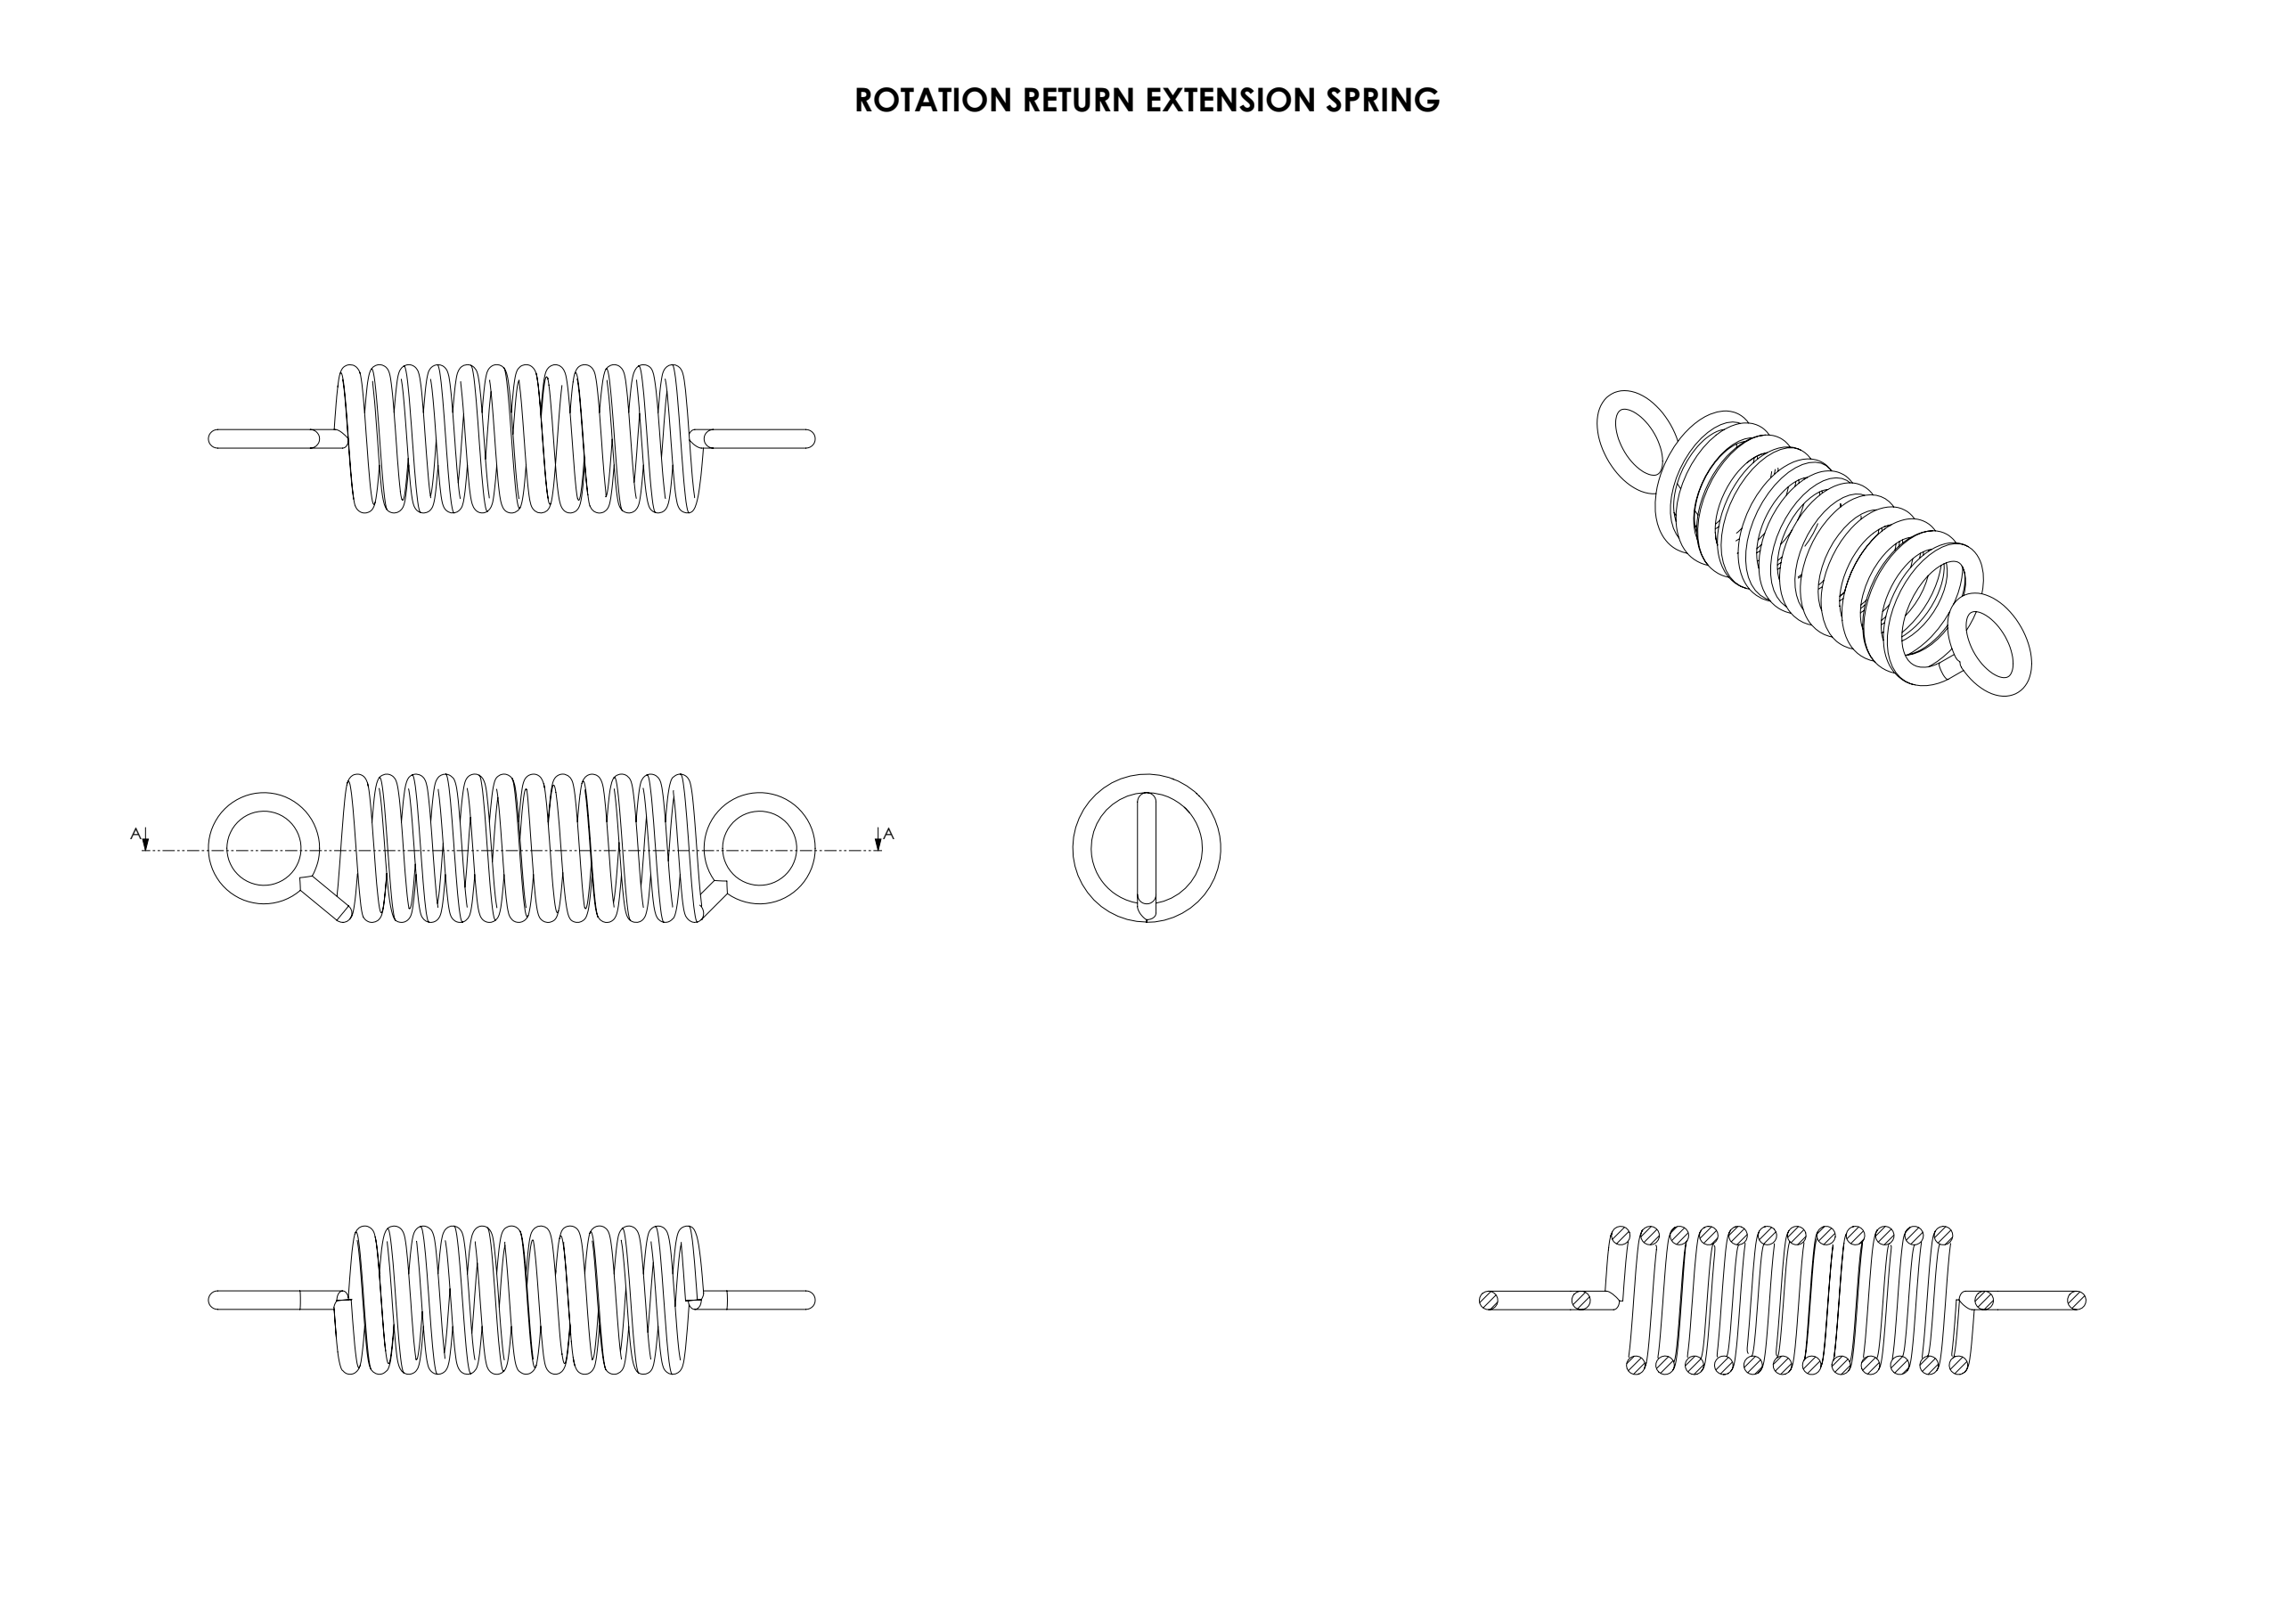
ISO-10303-21;
HEADER;
/* Generated by software containing ST-Developer
 * from STEP Tools, Inc. (www.steptools.com) 
 */

FILE_DESCRIPTION(
/* description */ (''),
/* implementation_level */ '2;1');

FILE_NAME(
/* name */ '16_Rotation_Return_Extension_Spring.step',
/* time_stamp */ '2026-10-21T01:56:51-07:00',
/* author */ (''),
/* organization */ (''),
/* preprocessor_version */ 'ST-DEVELOPER v20.2',
/* originating_system */ 'Autodesk Translation Framework v15.15.0.0',
/* authorisation */ '');

FILE_SCHEMA (('AUTOMOTIVE_DESIGN { 1 0 10303 214 3 1 1 }'));
ENDSEC;

DATA;
#10=MECHANICAL_DESIGN_GEOMETRIC_PRESENTATION_REPRESENTATION('',(#274),#82384);
#157=TOROIDAL_SURFACE('',#31771,2.,0.4);
#158=TOROIDAL_SURFACE('',#31779,2.,0.4);
#236=SHAPE_REPRESENTATION_RELATIONSHIP('SRR','None',#82470,#255);
#255=ADVANCED_BREP_SHAPE_REPRESENTATION('',(#293),#82369);
#274=STYLED_ITEM('',(#82631),#293);
#293=MANIFOLD_SOLID_BREP('Body1',#30665);
#418=B_SPLINE_SURFACE_WITH_KNOTS('',3,3,((#45016,#45017,#45018,#45019,#45020,
#45021,#45022,#45023,#45024,#45025,#45026,#45027,#45028,#45029,#45030,#45031,
#45032,#45033,#45034,#45035,#45036,#45037,#45038,#45039,#45040,#45041,#45042,
#45043,#45044,#45045,#45046,#45047,#45048,#45049,#45050,#45051,#45052,#45053,
#45054,#45055,#45056,#45057,#45058,#45059,#45060,#45061,#45062,#45063,#45064,
#45065,#45066,#45067,#45068,#45069,#45070,#45071,#45072,#45073,#45074,#45075,
#45076,#45077,#45078,#45079,#45080,#45081,#45082,#45083,#45084,#45085,#45086,
#45087,#45088,#45089,#45090,#45091,#45092,#45093,#45094,#45095,#45096,#45097,
#45098,#45099,#45100,#45101,#45102,#45103,#45104,#45105,#45106,#45107,#45108,
#45109,#45110,#45111,#45112,#45113,#45114,#45115,#45116,#45117,#45118,#45119,
#45120,#45121,#45122,#45123,#45124,#45125,#45126,#45127,#45128,#45129,#45130,
#45131,#45132,#45133,#45134,#45135,#45136,#45137,#45138,#45139,#45140,#45141,
#45142),(#45143,#45144,#45145,#45146,#45147,#45148,#45149,#45150,#45151,
#45152,#45153,#45154,#45155,#45156,#45157,#45158,#45159,#45160,#45161,#45162,
#45163,#45164,#45165,#45166,#45167,#45168,#45169,#45170,#45171,#45172,#45173,
#45174,#45175,#45176,#45177,#45178,#45179,#45180,#45181,#45182,#45183,#45184,
#45185,#45186,#45187,#45188,#45189,#45190,#45191,#45192,#45193,#45194,#45195,
#45196,#45197,#45198,#45199,#45200,#45201,#45202,#45203,#45204,#45205,#45206,
#45207,#45208,#45209,#45210,#45211,#45212,#45213,#45214,#45215,#45216,#45217,
#45218,#45219,#45220,#45221,#45222,#45223,#45224,#45225,#45226,#45227,#45228,
#45229,#45230,#45231,#45232,#45233,#45234,#45235,#45236,#45237,#45238,#45239,
#45240,#45241,#45242,#45243,#45244,#45245,#45246,#45247,#45248,#45249,#45250,
#45251,#45252,#45253,#45254,#45255,#45256,#45257,#45258,#45259,#45260,#45261,
#45262,#45263,#45264,#45265,#45266,#45267,#45268,#45269),(#45270,#45271,
#45272,#45273,#45274,#45275,#45276,#45277,#45278,#45279,#45280,#45281,#45282,
#45283,#45284,#45285,#45286,#45287,#45288,#45289,#45290,#45291,#45292,#45293,
#45294,#45295,#45296,#45297,#45298,#45299,#45300,#45301,#45302,#45303,#45304,
#45305,#45306,#45307,#45308,#45309,#45310,#45311,#45312,#45313,#45314,#45315,
#45316,#45317,#45318,#45319,#45320,#45321,#45322,#45323,#45324,#45325,#45326,
#45327,#45328,#45329,#45330,#45331,#45332,#45333,#45334,#45335,#45336,#45337,
#45338,#45339,#45340,#45341,#45342,#45343,#45344,#45345,#45346,#45347,#45348,
#45349,#45350,#45351,#45352,#45353,#45354,#45355,#45356,#45357,#45358,#45359,
#45360,#45361,#45362,#45363,#45364,#45365,#45366,#45367,#45368,#45369,#45370,
#45371,#45372,#45373,#45374,#45375,#45376,#45377,#45378,#45379,#45380,#45381,
#45382,#45383,#45384,#45385,#45386,#45387,#45388,#45389,#45390,#45391,#45392,
#45393,#45394,#45395,#45396),(#45397,#45398,#45399,#45400,#45401,#45402,
#45403,#45404,#45405,#45406,#45407,#45408,#45409,#45410,#45411,#45412,#45413,
#45414,#45415,#45416,#45417,#45418,#45419,#45420,#45421,#45422,#45423,#45424,
#45425,#45426,#45427,#45428,#45429,#45430,#45431,#45432,#45433,#45434,#45435,
#45436,#45437,#45438,#45439,#45440,#45441,#45442,#45443,#45444,#45445,#45446,
#45447,#45448,#45449,#45450,#45451,#45452,#45453,#45454,#45455,#45456,#45457,
#45458,#45459,#45460,#45461,#45462,#45463,#45464,#45465,#45466,#45467,#45468,
#45469,#45470,#45471,#45472,#45473,#45474,#45475,#45476,#45477,#45478,#45479,
#45480,#45481,#45482,#45483,#45484,#45485,#45486,#45487,#45488,#45489,#45490,
#45491,#45492,#45493,#45494,#45495,#45496,#45497,#45498,#45499,#45500,#45501,
#45502,#45503,#45504,#45505,#45506,#45507,#45508,#45509,#45510,#45511,#45512,
#45513,#45514,#45515,#45516,#45517,#45518,#45519,#45520,#45521,#45522,#45523),
(#45524,#45525,#45526,#45527,#45528,#45529,#45530,#45531,#45532,#45533,
#45534,#45535,#45536,#45537,#45538,#45539,#45540,#45541,#45542,#45543,#45544,
#45545,#45546,#45547,#45548,#45549,#45550,#45551,#45552,#45553,#45554,#45555,
#45556,#45557,#45558,#45559,#45560,#45561,#45562,#45563,#45564,#45565,#45566,
#45567,#45568,#45569,#45570,#45571,#45572,#45573,#45574,#45575,#45576,#45577,
#45578,#45579,#45580,#45581,#45582,#45583,#45584,#45585,#45586,#45587,#45588,
#45589,#45590,#45591,#45592,#45593,#45594,#45595,#45596,#45597,#45598,#45599,
#45600,#45601,#45602,#45603,#45604,#45605,#45606,#45607,#45608,#45609,#45610,
#45611,#45612,#45613,#45614,#45615,#45616,#45617,#45618,#45619,#45620,#45621,
#45622,#45623,#45624,#45625,#45626,#45627,#45628,#45629,#45630,#45631,#45632,
#45633,#45634,#45635,#45636,#45637,#45638,#45639,#45640,#45641,#45642,#45643,
#45644,#45645,#45646,#45647,#45648,#45649,#45650),(#45651,#45652,#45653,
#45654,#45655,#45656,#45657,#45658,#45659,#45660,#45661,#45662,#45663,#45664,
#45665,#45666,#45667,#45668,#45669,#45670,#45671,#45672,#45673,#45674,#45675,
#45676,#45677,#45678,#45679,#45680,#45681,#45682,#45683,#45684,#45685,#45686,
#45687,#45688,#45689,#45690,#45691,#45692,#45693,#45694,#45695,#45696,#45697,
#45698,#45699,#45700,#45701,#45702,#45703,#45704,#45705,#45706,#45707,#45708,
#45709,#45710,#45711,#45712,#45713,#45714,#45715,#45716,#45717,#45718,#45719,
#45720,#45721,#45722,#45723,#45724,#45725,#45726,#45727,#45728,#45729,#45730,
#45731,#45732,#45733,#45734,#45735,#45736,#45737,#45738,#45739,#45740,#45741,
#45742,#45743,#45744,#45745,#45746,#45747,#45748,#45749,#45750,#45751,#45752,
#45753,#45754,#45755,#45756,#45757,#45758,#45759,#45760,#45761,#45762,#45763,
#45764,#45765,#45766,#45767,#45768,#45769,#45770,#45771,#45772,#45773,#45774,
#45775,#45776,#45777),(#45778,#45779,#45780,#45781,#45782,#45783,#45784,
#45785,#45786,#45787,#45788,#45789,#45790,#45791,#45792,#45793,#45794,#45795,
#45796,#45797,#45798,#45799,#45800,#45801,#45802,#45803,#45804,#45805,#45806,
#45807,#45808,#45809,#45810,#45811,#45812,#45813,#45814,#45815,#45816,#45817,
#45818,#45819,#45820,#45821,#45822,#45823,#45824,#45825,#45826,#45827,#45828,
#45829,#45830,#45831,#45832,#45833,#45834,#45835,#45836,#45837,#45838,#45839,
#45840,#45841,#45842,#45843,#45844,#45845,#45846,#45847,#45848,#45849,#45850,
#45851,#45852,#45853,#45854,#45855,#45856,#45857,#45858,#45859,#45860,#45861,
#45862,#45863,#45864,#45865,#45866,#45867,#45868,#45869,#45870,#45871,#45872,
#45873,#45874,#45875,#45876,#45877,#45878,#45879,#45880,#45881,#45882,#45883,
#45884,#45885,#45886,#45887,#45888,#45889,#45890,#45891,#45892,#45893,#45894,
#45895,#45896,#45897,#45898,#45899,#45900,#45901,#45902,#45903,#45904),
(#45905,#45906,#45907,#45908,#45909,#45910,#45911,#45912,#45913,#45914,
#45915,#45916,#45917,#45918,#45919,#45920,#45921,#45922,#45923,#45924,#45925,
#45926,#45927,#45928,#45929,#45930,#45931,#45932,#45933,#45934,#45935,#45936,
#45937,#45938,#45939,#45940,#45941,#45942,#45943,#45944,#45945,#45946,#45947,
#45948,#45949,#45950,#45951,#45952,#45953,#45954,#45955,#45956,#45957,#45958,
#45959,#45960,#45961,#45962,#45963,#45964,#45965,#45966,#45967,#45968,#45969,
#45970,#45971,#45972,#45973,#45974,#45975,#45976,#45977,#45978,#45979,#45980,
#45981,#45982,#45983,#45984,#45985,#45986,#45987,#45988,#45989,#45990,#45991,
#45992,#45993,#45994,#45995,#45996,#45997,#45998,#45999,#46000,#46001,#46002,
#46003,#46004,#46005,#46006,#46007,#46008,#46009,#46010,#46011,#46012,#46013,
#46014,#46015,#46016,#46017,#46018,#46019,#46020,#46021,#46022,#46023,#46024,
#46025,#46026,#46027,#46028,#46029,#46030,#46031),(#46032,#46033,#46034,
#46035,#46036,#46037,#46038,#46039,#46040,#46041,#46042,#46043,#46044,#46045,
#46046,#46047,#46048,#46049,#46050,#46051,#46052,#46053,#46054,#46055,#46056,
#46057,#46058,#46059,#46060,#46061,#46062,#46063,#46064,#46065,#46066,#46067,
#46068,#46069,#46070,#46071,#46072,#46073,#46074,#46075,#46076,#46077,#46078,
#46079,#46080,#46081,#46082,#46083,#46084,#46085,#46086,#46087,#46088,#46089,
#46090,#46091,#46092,#46093,#46094,#46095,#46096,#46097,#46098,#46099,#46100,
#46101,#46102,#46103,#46104,#46105,#46106,#46107,#46108,#46109,#46110,#46111,
#46112,#46113,#46114,#46115,#46116,#46117,#46118,#46119,#46120,#46121,#46122,
#46123,#46124,#46125,#46126,#46127,#46128,#46129,#46130,#46131,#46132,#46133,
#46134,#46135,#46136,#46137,#46138,#46139,#46140,#46141,#46142,#46143,#46144,
#46145,#46146,#46147,#46148,#46149,#46150,#46151,#46152,#46153,#46154,#46155,
#46156,#46157,#46158),(#46159,#46160,#46161,#46162,#46163,#46164,#46165,
#46166,#46167,#46168,#46169,#46170,#46171,#46172,#46173,#46174,#46175,#46176,
#46177,#46178,#46179,#46180,#46181,#46182,#46183,#46184,#46185,#46186,#46187,
#46188,#46189,#46190,#46191,#46192,#46193,#46194,#46195,#46196,#46197,#46198,
#46199,#46200,#46201,#46202,#46203,#46204,#46205,#46206,#46207,#46208,#46209,
#46210,#46211,#46212,#46213,#46214,#46215,#46216,#46217,#46218,#46219,#46220,
#46221,#46222,#46223,#46224,#46225,#46226,#46227,#46228,#46229,#46230,#46231,
#46232,#46233,#46234,#46235,#46236,#46237,#46238,#46239,#46240,#46241,#46242,
#46243,#46244,#46245,#46246,#46247,#46248,#46249,#46250,#46251,#46252,#46253,
#46254,#46255,#46256,#46257,#46258,#46259,#46260,#46261,#46262,#46263,#46264,
#46265,#46266,#46267,#46268,#46269,#46270,#46271,#46272,#46273,#46274,#46275,
#46276,#46277,#46278,#46279,#46280,#46281,#46282,#46283,#46284,#46285)),
 .UNSPECIFIED.,.T.,.F.,.F.,(4,1,1,1,1,1,1,4),(4,1,1,1,1,1,1,1,1,1,1,1,1,
1,1,1,1,1,1,1,1,1,1,1,1,1,1,1,1,1,1,1,1,1,1,1,1,1,1,1,1,1,1,1,1,1,1,1,1,
1,1,1,1,1,1,1,1,1,1,1,1,1,1,1,1,1,1,1,1,1,1,1,1,1,1,1,1,1,1,1,1,1,1,1,1,
1,1,1,1,1,1,1,1,1,1,1,1,1,1,1,1,1,1,1,1,1,1,1,1,1,1,1,1,1,1,1,1,1,1,1,1,
1,1,1,4),(-3.14159265358979,-2.24399475256414,-1.34639685153848,-0.448798950512828,
0.448798950512828,1.34639685153848,2.24399475256414,3.14159265358979),(0.,
0.00446428571428571,0.00892857142857143,0.0178571428571429,0.0267857142857143,
0.0357142857142857,0.0446428571428571,0.0535714285714286,0.0625,0.0714285714285714,
0.0803571428571428,0.0892857142857143,0.0982142857142857,0.107142857142857,
0.116071428571429,0.125,0.129464285714286,0.133928571428571,0.138392857142857,
0.142857142857143,0.151785714285714,0.160714285714286,0.169642857142857,
0.178571428571429,0.1875,0.196428571428571,0.205357142857143,0.214285714285714,
0.223214285714286,0.232142857142857,0.241071428571429,0.25,0.258928571428571,
0.267857142857143,0.276785714285714,0.285714285714286,0.294642857142857,
0.303571428571429,0.3125,0.321428571428571,0.330357142857143,0.339285714285714,
0.348214285714286,0.357142857142857,0.366071428571428,0.375,0.383928571428571,
0.392857142857143,0.401785714285714,0.410714285714286,0.419642857142857,
0.428571428571429,0.4375,0.446428571428571,0.455357142857143,0.464285714285714,
0.473214285714286,0.482142857142857,0.494047619047619,0.5,0.504464285714286,
0.508928571428571,0.517857142857143,0.526785714285714,0.535714285714286,
0.544642857142857,0.553571428571429,0.5625,0.571428571428571,0.580357142857143,
0.589285714285714,0.598214285714286,0.607142857142857,0.616071428571429,
0.625,0.633928571428571,0.642857142857143,0.647321428571428,0.651785714285714,
0.660714285714286,0.666666666666667,0.678571428571428,0.6796875,0.680803571428571,
0.6875,0.696428571428571,0.705357142857143,0.714285714285714,0.726190476190476,
0.735119047619047,0.738095238095238,0.75,0.761904761904762,0.76984126984127,
0.777777777777778,0.785714285714286,0.793650793650794,0.801587301587302,
0.809523809523809,0.81547619047619,0.821428571428571,0.827380952380952,
0.830357142857143,0.833333333333333,0.839285714285714,0.845238095238095,
0.851190476190476,0.857142857142857,0.866071428571429,0.875,0.883928571428571,
0.892857142857143,0.901785714285714,0.910714285714286,0.919642857142857,
0.928571428571429,0.9375,0.946428571428571,0.955357142857143,0.964285714285714,
0.973214285714286,0.982142857142857,0.991071428571429,0.995535714285714,
1.),.UNSPECIFIED.);
#546=CYLINDRICAL_SURFACE('',#31767,0.4);
#547=CYLINDRICAL_SURFACE('',#31776,0.4);
#1421=CIRCLE('',#31768,0.4);
#1422=CIRCLE('',#31769,0.4);
#1423=CIRCLE('',#31772,0.4);
#1424=CIRCLE('',#31773,1.6);
#1425=CIRCLE('',#31775,0.4);
#1426=CIRCLE('',#31777,0.4);
#1427=CIRCLE('',#31780,0.4);
#1428=CIRCLE('',#31781,1.6);
#1429=CIRCLE('',#31783,0.4);
#2316=B_SPLINE_CURVE_WITH_KNOTS('',3,(#44822,#44823,#44824,#44825),
 .UNSPECIFIED.,.F.,.F.,(4,4),(-0.00278496917063749,0.000381985128916583),
 .UNSPECIFIED.);
#2317=B_SPLINE_CURVE_WITH_KNOTS('',3,(#44827,#44828,#44829,#44830,#44831,
#44832,#44833,#44834,#44835,#44836,#44837,#44838,#44839,#44840,#44841,#44842,
#44843,#44844,#44845,#44846,#44847,#44848),.UNSPECIFIED.,.F.,.F.,(4,2,2,
2,2,2,2,2,2,2,4),(-0.17876393636429,-0.178279109643944,-0.157081929142902,
-0.136547654157445,-0.114535014767487,-0.0983347050072544,-0.0847433634153561,
-0.0709327535553801,-0.0541499330631514,-0.0308889104943535,-0.00278496917063749),
 .UNSPECIFIED.);
#2318=B_SPLINE_CURVE_WITH_KNOTS('',3,(#44854,#44855,#44856,#44857,#44858,
#44859,#44860,#44861,#44862,#44863,#44864,#44865,#44866,#44867,#44868,#44869,
#44870,#44871,#44872,#44873,#44874,#44875,#44876,#44877,#44878,#44879),
 .UNSPECIFIED.,.F.,.F.,(4,2,2,2,2,2,2,2,2,2,2,2,4),(-0.149765769623311,
-0.149414895756082,-0.132671826505775,-0.114429386512108,-0.0992899556088679,
-0.0866980728560365,-0.074707447877953,-0.0627168228998696,-0.0501249401470389,
-0.0349855092437845,-0.0167430692500659,0.,0.000350873867280196),
 .UNSPECIFIED.);
#2319=B_SPLINE_CURVE_WITH_KNOTS('',3,(#44880,#44881,#44882,#44883,#44884,
#44885,#44886,#44887,#44888,#44889,#44890,#44891,#44892,#44893,#44894,#44895,
#44896,#44897,#44898,#44899,#44900,#44901,#44902,#44903,#44904,#44905),
 .UNSPECIFIED.,.F.,.F.,(4,2,2,2,2,2,2,2,2,2,2,2,4),(-0.149765769607808,
-0.149414895740571,-0.132671826492017,-0.114429386500231,-0.0992899555985793,
-0.086698072847082,-0.0747074478702766,-0.0627168228934715,-0.0501249401419783,
-0.0349855092403365,-0.0167430692485508,0.,0.000350873867236666),
 .UNSPECIFIED.);
#2320=B_SPLINE_CURVE_WITH_KNOTS('',3,(#44918,#44919,#44920,#44921,#44922,
#44923,#44924,#44925),.UNSPECIFIED.,.F.,.F.,(4,2,2,4),(-0.12173108833567,
-0.113308899129218,-0.097236345543046,-0.0881725331804662),
 .UNSPECIFIED.);
#2321=B_SPLINE_CURVE_WITH_KNOTS('',3,(#44927,#44928,#44929,#44930,#44931,
#44932,#44933,#44934,#44935,#44936),.UNSPECIFIED.,.F.,.F.,(4,2,2,2,4),(-0.177908635507065,
-0.177425299894269,-0.155806602995727,-0.134924086342148,-0.12173108833567),
 .UNSPECIFIED.);
#2322=B_SPLINE_CURVE_WITH_KNOTS('',3,(#44939,#44940,#44941,#44942,#44943,
#44944,#44945,#44946,#44947,#44948,#44949,#44950,#44951,#44952),
 .UNSPECIFIED.,.F.,.F.,(4,2,2,2,2,2,4),(-0.0881725331804662,-0.0836000761729691,
-0.069663721232867,-0.0537475177849022,-0.0307021203616524,0.,0.000380437960906122),
 .UNSPECIFIED.);
#2323=B_SPLINE_CURVE_WITH_KNOTS('',3,(#44956,#44957,#44958,#44959,#44960,
#44961,#44962,#44963,#44964,#44965,#44966,#44967,#44968,#44969,#44970,#44971,
#44972,#44973,#44974,#44975,#44976,#44977,#44978,#44979,#44980,#44981),
 .UNSPECIFIED.,.F.,.F.,(4,2,2,2,2,2,2,2,2,2,2,2,4),(-0.149766416121483,
-0.149416311689899,-0.132681110939406,-0.11446620080775,-0.0993072249168199,
-0.0867023299576758,-0.074708155848574,-0.0627139817394723,-0.0501090867803249,
-0.0349501108893815,-0.0167352007577163,0.,0.000350104430293171),
 .UNSPECIFIED.);
#2324=B_SPLINE_CURVE_WITH_KNOTS('',3,(#44982,#44983,#44984,#44985,#44986,
#44987,#44988,#44989,#44990,#44991,#44992,#44993,#44994,#44995,#44996,#44997,
#44998,#44999,#45000,#45001,#45002,#45003,#45004,#45005,#45006,#45007),
 .UNSPECIFIED.,.F.,.F.,(4,2,2,2,2,2,2,2,2,2,2,2,4),(-0.149766416599849,
-0.149416312168387,-0.132681111357522,-0.114466201167421,-0.0993072252278703,
-0.0867023302283183,-0.0747081560807638,-0.0627139819332097,-0.0501090869336602,
-0.0349501109941116,-0.0167352008040167,0.,0.000350104432701244),
 .UNSPECIFIED.);
#2325=B_SPLINE_CURVE_WITH_KNOTS('',3,(#46286,#46287,#46288,#46289,#46290,
#46291,#46292,#46293,#46294,#46295,#46296,#46297,#46298,#46299,#46300,#46301,
#46302,#46303,#46304,#46305,#46306,#46307,#46308,#46309,#46310,#46311,#46312,
#46313,#46314,#46315,#46316,#46317,#46318,#46319,#46320,#46321,#46322,#46323,
#46324,#46325,#46326,#46327,#46328,#46329,#46330,#46331,#46332,#46333,#46334,
#46335,#46336,#46337,#46338,#46339,#46340,#46341,#46342,#46343,#46344,#46345,
#46346,#46347,#46348,#46349,#46350,#46351,#46352,#46353,#46354,#46355,#46356,
#46357,#46358,#46359,#46360,#46361,#46362,#46363,#46364,#46365,#46366,#46367,
#46368,#46369,#46370,#46371,#46372,#46373,#46374,#46375,#46376,#46377,#46378,
#46379,#46380,#46381,#46382,#46383,#46384,#46385,#46386,#46387,#46388,#46389,
#46390,#46391,#46392,#46393,#46394,#46395,#46396,#46397,#46398,#46399,#46400,
#46401,#46402,#46403,#46404,#46405,#46406,#46407,#46408,#46409,#46410,#46411,
#46412),.UNSPECIFIED.,.F.,.F.,(4,1,1,1,1,1,1,1,1,1,1,1,1,1,1,1,1,1,1,1,
1,1,1,1,1,1,1,1,1,1,1,1,1,1,1,1,1,1,1,1,1,1,1,1,1,1,1,1,1,1,1,1,1,1,1,1,
1,1,1,1,1,1,1,1,1,1,1,1,1,1,1,1,1,1,1,1,1,1,1,1,1,1,1,1,1,1,1,1,1,1,1,1,
1,1,1,1,1,1,1,1,1,1,1,1,1,1,1,1,1,1,1,1,1,1,1,1,1,1,1,1,1,1,1,1,4),(0.00137832727077589,
0.00446428571428571,0.00892857142857143,0.0178571428571429,0.0267857142857143,
0.0357142857142857,0.0446428571428571,0.0535714285714286,0.0625,0.0714285714285714,
0.0803571428571428,0.0892857142857143,0.0982142857142857,0.107142857142857,
0.116071428571429,0.125,0.129464285714286,0.133928571428571,0.138392857142857,
0.142857142857143,0.151785714285714,0.160714285714286,0.169642857142857,
0.178571428571429,0.1875,0.196428571428571,0.205357142857143,0.214285714285714,
0.223214285714286,0.232142857142857,0.241071428571429,0.25,0.258928571428571,
0.267857142857143,0.276785714285714,0.285714285714286,0.294642857142857,
0.303571428571429,0.3125,0.321428571428571,0.330357142857143,0.339285714285714,
0.348214285714286,0.357142857142857,0.366071428571428,0.375,0.383928571428571,
0.392857142857143,0.401785714285714,0.410714285714286,0.419642857142857,
0.428571428571429,0.4375,0.446428571428571,0.455357142857143,0.464285714285714,
0.473214285714286,0.482142857142857,0.494047619047619,0.5,0.504464285714286,
0.508928571428571,0.517857142857143,0.526785714285714,0.535714285714286,
0.544642857142857,0.553571428571429,0.5625,0.571428571428571,0.580357142857143,
0.589285714285714,0.598214285714286,0.607142857142857,0.616071428571429,
0.625,0.633928571428571,0.642857142857143,0.647321428571428,0.651785714285714,
0.660714285714286,0.666666666666667,0.678571428571428,0.6796875,0.680803571428571,
0.6875,0.696428571428571,0.705357142857143,0.714285714285714,0.726190476190476,
0.735119047619047,0.738095238095238,0.75,0.761904761904762,0.76984126984127,
0.777777777777778,0.785714285714286,0.793650793650794,0.801587301587302,
0.809523809523809,0.81547619047619,0.821428571428571,0.827380952380952,
0.830357142857143,0.833333333333333,0.839285714285714,0.845238095238095,
0.851190476190476,0.857142857142857,0.866071428571429,0.875,0.883928571428571,
0.892857142857143,0.901785714285714,0.910714285714286,0.919642857142857,
0.928571428571429,0.9375,0.946428571428571,0.955357142857143,0.964285714285714,
0.973214285714286,0.982142857142857,0.991071428571429,0.995535714285714,
0.999890109193126),.UNSPECIFIED.);
#3443=FACE_BOUND('',#6091,.T.);
#3444=FACE_BOUND('',#6096,.T.);
#4173=FACE_OUTER_BOUND('',#6088,.T.);
#4174=FACE_OUTER_BOUND('',#6089,.T.);
#4175=FACE_OUTER_BOUND('',#6090,.T.);
#4176=FACE_OUTER_BOUND('',#6092,.T.);
#4177=FACE_OUTER_BOUND('',#6093,.T.);
#4178=FACE_OUTER_BOUND('',#6094,.T.);
#4179=FACE_OUTER_BOUND('',#6095,.T.);
#4180=FACE_OUTER_BOUND('',#6097,.T.);
#4181=FACE_OUTER_BOUND('',#6098,.T.);
#6088=EDGE_LOOP('',(#22101,#22102,#22103,#22104,#22105,#22106,#22107,#22108));
#6089=EDGE_LOOP('',(#22109,#22110,#22111));
#6090=EDGE_LOOP('',(#22112,#22113,#22114,#22115));
#6091=EDGE_LOOP('',(#22116,#22117));
#6092=EDGE_LOOP('',(#22118,#22119));
#6093=EDGE_LOOP('',(#22120,#22121,#22122,#22123,#22124,#22125,#22126,#22127));
#6094=EDGE_LOOP('',(#22128,#22129));
#6095=EDGE_LOOP('',(#22130,#22131,#22132,#22133));
#6096=EDGE_LOOP('',(#22134,#22135));
#6097=EDGE_LOOP('',(#22136,#22137));
#6098=EDGE_LOOP('',(#22138,#22139,#22140,#22141,#22142,#22143,#22144,#22145,
#22146));
#8172=LINE('',#44852,#10478);
#8173=LINE('',#44908,#10479);
#8174=LINE('',#44954,#10480);
#8175=LINE('',#45009,#10481);
#10478=VECTOR('',#35961,0.4);
#10479=VECTOR('',#35966,10.);
#10480=VECTOR('',#35981,0.4);
#10481=VECTOR('',#35984,10.);
#12869=VERTEX_POINT('',#44820);
#12870=VERTEX_POINT('',#44821);
#12871=VERTEX_POINT('',#44826);
#12872=VERTEX_POINT('',#44849);
#12873=VERTEX_POINT('',#44851);
#12874=VERTEX_POINT('',#44853);
#12875=VERTEX_POINT('',#44910);
#12876=VERTEX_POINT('',#44916);
#12877=VERTEX_POINT('',#44917);
#12878=VERTEX_POINT('',#44926);
#12879=VERTEX_POINT('',#44937);
#12880=VERTEX_POINT('',#44953);
#12881=VERTEX_POINT('',#44955);
#12882=VERTEX_POINT('',#45011);
#16272=EDGE_CURVE('',#12869,#12870,#2316,.T.);
#16273=EDGE_CURVE('',#12871,#12869,#2317,.T.);
#16274=EDGE_CURVE('',#12872,#12871,#1421,.T.);
#16275=EDGE_CURVE('',#12872,#12873,#8172,.T.);
#16276=EDGE_CURVE('',#12874,#12873,#2318,.T.);
#16277=EDGE_CURVE('',#12873,#12874,#2319,.T.);
#16278=EDGE_CURVE('',#12870,#12872,#1422,.T.);
#16279=EDGE_CURVE('',#12870,#12871,#8173,.T.);
#16280=EDGE_CURVE('',#12875,#12875,#1423,.T.);
#16281=EDGE_CURVE('',#12875,#12875,#1424,.T.);
#16282=EDGE_CURVE('',#12871,#12870,#1425,.T.);
#16283=EDGE_CURVE('',#12876,#12877,#2320,.T.);
#16284=EDGE_CURVE('',#12878,#12876,#2321,.T.);
#16285=EDGE_CURVE('',#12879,#12878,#1426,.T.);
#16286=EDGE_CURVE('',#12877,#12879,#2322,.T.);
#16287=EDGE_CURVE('',#12877,#12880,#8174,.T.);
#16288=EDGE_CURVE('',#12881,#12880,#2323,.T.);
#16289=EDGE_CURVE('',#12880,#12881,#2324,.T.);
#16290=EDGE_CURVE('',#12879,#12878,#8175,.T.);
#16291=EDGE_CURVE('',#12882,#12882,#1427,.T.);
#16292=EDGE_CURVE('',#12882,#12882,#1428,.T.);
#16293=EDGE_CURVE('',#12879,#12878,#1429,.T.);
#16294=EDGE_CURVE('',#12876,#12869,#2325,.T.);
#22101=ORIENTED_EDGE('',*,*,#16272,.F.);
#22102=ORIENTED_EDGE('',*,*,#16273,.F.);
#22103=ORIENTED_EDGE('',*,*,#16274,.F.);
#22104=ORIENTED_EDGE('',*,*,#16275,.T.);
#22105=ORIENTED_EDGE('',*,*,#16276,.F.);
#22106=ORIENTED_EDGE('',*,*,#16277,.F.);
#22107=ORIENTED_EDGE('',*,*,#16275,.F.);
#22108=ORIENTED_EDGE('',*,*,#16278,.F.);
#22109=ORIENTED_EDGE('',*,*,#16279,.F.);
#22110=ORIENTED_EDGE('',*,*,#16278,.T.);
#22111=ORIENTED_EDGE('',*,*,#16274,.T.);
#22112=ORIENTED_EDGE('',*,*,#16280,.F.);
#22113=ORIENTED_EDGE('',*,*,#16281,.T.);
#22114=ORIENTED_EDGE('',*,*,#16280,.T.);
#22115=ORIENTED_EDGE('',*,*,#16281,.F.);
#22116=ORIENTED_EDGE('',*,*,#16276,.T.);
#22117=ORIENTED_EDGE('',*,*,#16277,.T.);
#22118=ORIENTED_EDGE('',*,*,#16279,.T.);
#22119=ORIENTED_EDGE('',*,*,#16282,.T.);
#22120=ORIENTED_EDGE('',*,*,#16283,.F.);
#22121=ORIENTED_EDGE('',*,*,#16284,.F.);
#22122=ORIENTED_EDGE('',*,*,#16285,.F.);
#22123=ORIENTED_EDGE('',*,*,#16286,.F.);
#22124=ORIENTED_EDGE('',*,*,#16287,.T.);
#22125=ORIENTED_EDGE('',*,*,#16288,.F.);
#22126=ORIENTED_EDGE('',*,*,#16289,.F.);
#22127=ORIENTED_EDGE('',*,*,#16287,.F.);
#22128=ORIENTED_EDGE('',*,*,#16290,.F.);
#22129=ORIENTED_EDGE('',*,*,#16285,.T.);
#22130=ORIENTED_EDGE('',*,*,#16291,.F.);
#22131=ORIENTED_EDGE('',*,*,#16292,.T.);
#22132=ORIENTED_EDGE('',*,*,#16291,.T.);
#22133=ORIENTED_EDGE('',*,*,#16292,.F.);
#22134=ORIENTED_EDGE('',*,*,#16288,.T.);
#22135=ORIENTED_EDGE('',*,*,#16289,.T.);
#22136=ORIENTED_EDGE('',*,*,#16290,.T.);
#22137=ORIENTED_EDGE('',*,*,#16293,.F.);
#22138=ORIENTED_EDGE('',*,*,#16272,.T.);
#22139=ORIENTED_EDGE('',*,*,#16282,.F.);
#22140=ORIENTED_EDGE('',*,*,#16273,.T.);
#22141=ORIENTED_EDGE('',*,*,#16294,.F.);
#22142=ORIENTED_EDGE('',*,*,#16283,.T.);
#22143=ORIENTED_EDGE('',*,*,#16286,.T.);
#22144=ORIENTED_EDGE('',*,*,#16293,.T.);
#22145=ORIENTED_EDGE('',*,*,#16284,.T.);
#22146=ORIENTED_EDGE('',*,*,#16294,.T.);
#28309=PLANE('',#31770);
#28310=PLANE('',#31774);
#28311=PLANE('',#31778);
#28312=PLANE('',#31782);
#29501=ADVANCED_FACE('',(#4173),#546,.T.);
#29502=ADVANCED_FACE('',(#4174),#28309,.T.);
#29503=ADVANCED_FACE('',(#4175,#3443),#157,.T.);
#29504=ADVANCED_FACE('',(#4176),#28310,.T.);
#29505=ADVANCED_FACE('',(#4177),#547,.T.);
#29506=ADVANCED_FACE('',(#4178),#28311,.T.);
#29507=ADVANCED_FACE('',(#4179,#3444),#158,.T.);
#29508=ADVANCED_FACE('',(#4180),#28312,.F.);
#29509=ADVANCED_FACE('',(#4181),#418,.T.);
#30665=CLOSED_SHELL('',(#29501,#29502,#29503,#29504,#29505,#29506,#29507,
#29508,#29509));
#31766=AXIS2_PLACEMENT_3D('',#44818,#35955,#35956);
#31767=AXIS2_PLACEMENT_3D('',#44819,#35957,#35958);
#31768=AXIS2_PLACEMENT_3D('',#44850,#35959,#35960);
#31769=AXIS2_PLACEMENT_3D('',#44906,#35962,#35963);
#31770=AXIS2_PLACEMENT_3D('',#44907,#35964,#35965);
#31771=AXIS2_PLACEMENT_3D('',#44909,#35967,#35968);
#31772=AXIS2_PLACEMENT_3D('',#44911,#35969,#35970);
#31773=AXIS2_PLACEMENT_3D('',#44912,#35971,#35972);
#31774=AXIS2_PLACEMENT_3D('',#44913,#35973,#35974);
#31775=AXIS2_PLACEMENT_3D('',#44914,#35975,#35976);
#31776=AXIS2_PLACEMENT_3D('',#44915,#35977,#35978);
#31777=AXIS2_PLACEMENT_3D('',#44938,#35979,#35980);
#31778=AXIS2_PLACEMENT_3D('',#45008,#35982,#35983);
#31779=AXIS2_PLACEMENT_3D('',#45010,#35985,#35986);
#31780=AXIS2_PLACEMENT_3D('',#45012,#35987,#35988);
#31781=AXIS2_PLACEMENT_3D('',#45013,#35989,#35990);
#31782=AXIS2_PLACEMENT_3D('',#45014,#35991,#35992);
#31783=AXIS2_PLACEMENT_3D('',#45015,#35993,#35994);
#35955=DIRECTION('axis',(0.,0.,1.));
#35956=DIRECTION('refdir',(1.,0.,0.));
#35957=DIRECTION('center_axis',(-0.707106781186548,-0.707106781186548,0.));
#35958=DIRECTION('ref_axis',(-3.33066907387547E-16,3.33066907387547E-16,
1.));
#35959=DIRECTION('center_axis',(-0.707106781186548,-0.707106781186548,0.));
#35960=DIRECTION('ref_axis',(-3.33066907387547E-16,3.33066907387547E-16,
1.));
#35961=DIRECTION('',(0.707106781186548,0.707106781186548,0.));
#35962=DIRECTION('center_axis',(-0.707106781186548,-0.707106781186548,0.));
#35963=DIRECTION('ref_axis',(-3.33066907387547E-16,3.33066907387547E-16,
1.));
#35964=DIRECTION('center_axis',(-0.707106781186548,-0.707106781186548,0.));
#35965=DIRECTION('ref_axis',(-3.33066907387547E-16,3.33066907387547E-16,
1.));
#35966=DIRECTION('',(0.706176214723467,-0.706176214723467,0.0512865237432823));
#35967=DIRECTION('center_axis',(0.,0.,1.));
#35968=DIRECTION('ref_axis',(1.,0.,0.));
#35969=DIRECTION('center_axis',(0.,-1.,0.));
#35970=DIRECTION('ref_axis',(-1.,0.,0.));
#35971=DIRECTION('center_axis',(0.,0.,-1.));
#35972=DIRECTION('ref_axis',(1.,0.,0.));
#35973=DIRECTION('center_axis',(0.0706021761589144,-0.0018421410289849,
-0.997502851744322));
#35974=DIRECTION('ref_axis',(0.663761346011967,-0.746379469565852,0.0483586905424292));
#35975=DIRECTION('center_axis',(0.0706021761589144,-0.0018421410289849,
-0.997502851744322));
#35976=DIRECTION('ref_axis',(0.663761346011967,-0.746379469565852,0.0483586905424292));
#35977=DIRECTION('center_axis',(0.77193023561705,-0.635707252861099,0.));
#35978=DIRECTION('ref_axis',(3.20476749376334E-17,3.89150338528406E-17,
1.));
#35979=DIRECTION('center_axis',(0.77193023561705,-0.635707252861099,1.13428418954078E-16));
#35980=DIRECTION('ref_axis',(-5.55111512312578E-17,1.11022302462516E-16,
1.));
#35981=DIRECTION('',(-0.77193023561705,0.635707252861099,0.));
#35982=DIRECTION('center_axis',(0.77193023561705,-0.635707252861099,1.13428418954078E-16));
#35983=DIRECTION('ref_axis',(-5.55111512312578E-17,1.11022302462516E-16,
1.));
#35984=DIRECTION('',(-0.635023434538235,-0.771099884796429,-0.0463703057375958));
#35985=DIRECTION('center_axis',(0.,0.,1.));
#35986=DIRECTION('ref_axis',(1.,0.,0.));
#35987=DIRECTION('center_axis',(0.,-1.,0.));
#35988=DIRECTION('ref_axis',(-1.,0.,0.));
#35989=DIRECTION('center_axis',(0.,0.,-1.));
#35990=DIRECTION('ref_axis',(1.,0.,0.));
#35991=DIRECTION('center_axis',(0.070602176935317,0.00184214179195253,-0.99750285168796));
#35992=DIRECTION('ref_axis',(0.997163482507387,0.0260178454018302,0.0706262052951131));
#35993=DIRECTION('center_axis',(0.070602176935317,0.00184214179195253,-0.99750285168796));
#35994=DIRECTION('ref_axis',(0.997163482507387,0.0260178454018302,0.0706262052951131));
#44818=CARTESIAN_POINT('',(0.,0.,0.));
#44819=CARTESIAN_POINT('Origin',(-40.0142135623731,-80.4142135623731,20.));
#44820=CARTESIAN_POINT('',(-41.6670038745204,-81.5013243192465,20.0018221889518));
#44821=CARTESIAN_POINT('',(-41.6824373695361,-81.5175532542339,19.9794877782846));
#44822=CARTESIAN_POINT('Ctrl Pts',(-41.667003992987,-81.501323636858,20.0018258382422));
#44823=CARTESIAN_POINT('Ctrl Pts',(-41.6723036980297,-81.5065761360697,
19.9943901405908));
#44824=CARTESIAN_POINT('Ctrl Pts',(-41.6774508057097,-81.5119900511825,
19.9869413272942));
#44825=CARTESIAN_POINT('Ctrl Pts',(-41.6824371476317,-81.5175534133105,
19.9794877942845));
#44826=CARTESIAN_POINT('',(-41.1175295141106,-82.0824704858893,20.0205146094984));
#44827=CARTESIAN_POINT('Ctrl Pts',(-41.1175295141106,-82.0824704858894,
20.0205146094973));
#44828=CARTESIAN_POINT('Ctrl Pts',(-41.1169315617889,-82.0818012262451,
20.0214964568026));
#44829=CARTESIAN_POINT('Ctrl Pts',(-41.1163360655611,-82.0811293124528,
20.022477994219));
#44830=CARTESIAN_POINT('Ctrl Pts',(-41.0898149851225,-82.050962453584,20.0663587246604));
#44831=CARTESIAN_POINT('Ctrl Pts',(-41.0684925512851,-82.0163047514998,
20.1087879830725));
#44832=CARTESIAN_POINT('Ctrl Pts',(-41.0371790069056,-81.9399561963918,
20.1880837226203));
#44833=CARTESIAN_POINT('Ctrl Pts',(-41.026715172619,-81.8981742709483,20.2254321238237));
#44834=CARTESIAN_POINT('Ctrl Pts',(-41.017874801645,-81.8053693573189,20.2952495938576));
#44835=CARTESIAN_POINT('Ctrl Pts',(-41.0203629078659,-81.7532119643487,
20.3276528784673));
#44836=CARTESIAN_POINT('Ctrl Pts',(-41.0413539676923,-81.6607507752854,
20.3707052159476));
#44837=CARTESIAN_POINT('Ctrl Pts',(-41.0555000619675,-81.6208986488143,
20.3848443838584));
#44838=CARTESIAN_POINT('Ctrl Pts',(-41.093188372277,-81.5507282918097,20.3994995890491));
#44839=CARTESIAN_POINT('Ctrl Pts',(-41.1144544593006,-81.5206896773008,
20.401675192587));
#44840=CARTESIAN_POINT('Ctrl Pts',(-41.165653789439,-81.4669930646739,20.3956510376664));
#44841=CARTESIAN_POINT('Ctrl Pts',(-41.1944668468356,-81.4447737703187,
20.387440961117));
#44842=CARTESIAN_POINT('Ctrl Pts',(-41.2629514740271,-81.406840654893,20.3593672352608));
#44843=CARTESIAN_POINT('Ctrl Pts',(-41.3018885474464,-81.394495024668,20.3381091044114));
#44844=CARTESIAN_POINT('Ctrl Pts',(-41.3929538579519,-81.3809801263275,
20.2795382731015));
#44845=CARTESIAN_POINT('Ctrl Pts',(-41.4471194419021,-81.3855135588177,
20.2374603554904));
#44846=CARTESIAN_POINT('Ctrl Pts',(-41.5618160326496,-81.4200211943617,
20.1322968488021));
#44847=CARTESIAN_POINT('Ctrl Pts',(-41.6199733871036,-81.4547186766113,
20.0677665047026));
#44848=CARTESIAN_POINT('Ctrl Pts',(-41.6670038745197,-81.5013243192459,
20.0018221889509));
#44849=CARTESIAN_POINT('',(-41.4,-81.8,19.6));
#44850=CARTESIAN_POINT('Origin',(-41.4,-81.8,20.));
#44851=CARTESIAN_POINT('',(-40.0142135623731,-80.4142135623731,19.6));
#44852=CARTESIAN_POINT('',(-40.0142135623731,-80.4142135623731,19.6));
#44853=CARTESIAN_POINT('',(-40.0142135623731,-80.4142135623731,20.4));
#44854=CARTESIAN_POINT('Ctrl Pts',(-40.0142135623731,-80.4142135623731,
20.4));
#44855=CARTESIAN_POINT('Ctrl Pts',(-40.0142135623731,-80.4153831419304,
20.4));
#44856=CARTESIAN_POINT('Ctrl Pts',(-40.0142131996467,-80.4165527237652,
20.3999974351574));
#44857=CARTESIAN_POINT('Ctrl Pts',(-40.0141778904501,-80.4735319741397,
20.3997472920084));
#44858=CARTESIAN_POINT('Ctrl Pts',(-40.013302136999,-80.5295473343443,20.3936524317683));
#44859=CARTESIAN_POINT('Ctrl Pts',(-40.0100460838861,-80.6429937614698,
20.3672982573464));
#44860=CARTESIAN_POINT('Ctrl Pts',(-40.0075166610327,-80.7005682273989,
20.3457022349177));
#44861=CARTESIAN_POINT('Ctrl Pts',(-40.0022566529727,-80.7962497320611,
20.2899515263984));
#44862=CARTESIAN_POINT('Ctrl Pts',(-39.999637895333,-80.836023977406,20.2585158351079));
#44863=CARTESIAN_POINT('Ctrl Pts',(-39.9953022634654,-80.8963784968088,
20.1894129105366));
#44864=CARTESIAN_POINT('Ctrl Pts',(-39.9935403080928,-80.9187129635945,
20.1540514056522));
#44865=CARTESIAN_POINT('Ctrl Pts',(-39.991131445458,-80.9484928880337,20.0784645960831));
#44866=CARTESIAN_POINT('Ctrl Pts',(-39.9904773405935,-80.9561627655428,
20.039614799918));
#44867=CARTESIAN_POINT('Ctrl Pts',(-39.9904773405935,-80.9561627655428,
19.960385200082));
#44868=CARTESIAN_POINT('Ctrl Pts',(-39.991131445458,-80.9484928880337,19.9215354039169));
#44869=CARTESIAN_POINT('Ctrl Pts',(-39.9935403080928,-80.9187129635945,
19.8459485943478));
#44870=CARTESIAN_POINT('Ctrl Pts',(-39.9953022634654,-80.8963784968088,
19.8105870894634));
#44871=CARTESIAN_POINT('Ctrl Pts',(-39.999637895333,-80.8360239774059,19.741484164892));
#44872=CARTESIAN_POINT('Ctrl Pts',(-40.0022566529728,-80.796249732061,19.7100484736016));
#44873=CARTESIAN_POINT('Ctrl Pts',(-40.0075166610327,-80.7005682273989,
19.6542977650823));
#44874=CARTESIAN_POINT('Ctrl Pts',(-40.0100460838861,-80.6429937614698,
19.6327017426536));
#44875=CARTESIAN_POINT('Ctrl Pts',(-40.013302136999,-80.5295473343452,19.6063475682319));
#44876=CARTESIAN_POINT('Ctrl Pts',(-40.0141778904501,-80.473531974145,19.6002527079916));
#44877=CARTESIAN_POINT('Ctrl Pts',(-40.0142131996467,-80.4165527237649,
19.6000025648426));
#44878=CARTESIAN_POINT('Ctrl Pts',(-40.0142135623731,-80.4153831419307,
19.6));
#44879=CARTESIAN_POINT('Ctrl Pts',(-40.0142135623731,-80.4142135623731,
19.6));
#44880=CARTESIAN_POINT('Ctrl Pts',(-40.0142135623731,-80.4142135623731,
19.6));
#44881=CARTESIAN_POINT('Ctrl Pts',(-40.0153831419306,-80.4142135623731,
19.6));
#44882=CARTESIAN_POINT('Ctrl Pts',(-40.016552723765,-80.4142131996467,19.6000025648426));
#44883=CARTESIAN_POINT('Ctrl Pts',(-40.0735319741399,-80.4141778904502,
19.6002527079916));
#44884=CARTESIAN_POINT('Ctrl Pts',(-40.1295473343444,-80.413302136999,19.6063475682317));
#44885=CARTESIAN_POINT('Ctrl Pts',(-40.2429937614698,-80.4100460838861,
19.6327017426536));
#44886=CARTESIAN_POINT('Ctrl Pts',(-40.300568227399,-80.4075166610327,19.6542977650823));
#44887=CARTESIAN_POINT('Ctrl Pts',(-40.396249732061,-80.4022566529727,19.7100484736016));
#44888=CARTESIAN_POINT('Ctrl Pts',(-40.436023977406,-80.399637895333,19.741484164892));
#44889=CARTESIAN_POINT('Ctrl Pts',(-40.4963784968088,-80.3953022634654,
19.8105870894634));
#44890=CARTESIAN_POINT('Ctrl Pts',(-40.5187129635945,-80.3935403080928,
19.8459485943478));
#44891=CARTESIAN_POINT('Ctrl Pts',(-40.5484928880337,-80.391131445458,19.9215354039169));
#44892=CARTESIAN_POINT('Ctrl Pts',(-40.5561627655428,-80.3904773405935,
19.960385200082));
#44893=CARTESIAN_POINT('Ctrl Pts',(-40.5561627655428,-80.3904773405935,
20.039614799918));
#44894=CARTESIAN_POINT('Ctrl Pts',(-40.5484928880337,-80.391131445458,20.0784645960831));
#44895=CARTESIAN_POINT('Ctrl Pts',(-40.5187129635945,-80.3935403080928,
20.1540514056522));
#44896=CARTESIAN_POINT('Ctrl Pts',(-40.4963784968088,-80.3953022634654,
20.1894129105366));
#44897=CARTESIAN_POINT('Ctrl Pts',(-40.436023977406,-80.399637895333,20.258515835108));
#44898=CARTESIAN_POINT('Ctrl Pts',(-40.396249732061,-80.4022566529727,20.2899515263984));
#44899=CARTESIAN_POINT('Ctrl Pts',(-40.300568227399,-80.4075166610327,20.3457022349177));
#44900=CARTESIAN_POINT('Ctrl Pts',(-40.2429937614698,-80.4100460838861,
20.3672982573464));
#44901=CARTESIAN_POINT('Ctrl Pts',(-40.1295473343444,-80.413302136999,20.3936524317682));
#44902=CARTESIAN_POINT('Ctrl Pts',(-40.0735319741399,-80.4141778904502,
20.3997472920084));
#44903=CARTESIAN_POINT('Ctrl Pts',(-40.016552723765,-80.4142131996467,20.3999974351574));
#44904=CARTESIAN_POINT('Ctrl Pts',(-40.0153831419306,-80.4142135623731,
20.4));
#44905=CARTESIAN_POINT('Ctrl Pts',(-40.0142135623731,-80.4142135623731,
20.4));
#44906=CARTESIAN_POINT('Origin',(-41.4,-81.8,20.));
#44907=CARTESIAN_POINT('Origin',(-41.4,-81.8,20.));
#44908=CARTESIAN_POINT('',(-41.4,-81.8,20.));
#44909=CARTESIAN_POINT('Origin',(-38.6,-79.,20.));
#44910=CARTESIAN_POINT('',(-40.2,-79.,20.));
#44911=CARTESIAN_POINT('Origin',(-40.6,-79.,20.));
#44912=CARTESIAN_POINT('Origin',(-38.6,-79.,20.));
#44913=CARTESIAN_POINT('Origin',(-41.4,-81.8,20.));
#44914=CARTESIAN_POINT('Origin',(-41.4,-81.8,20.));
#44915=CARTESIAN_POINT('Origin',(-58.4561395287659,-80.2714145057222,20.));
#44916=CARTESIAN_POINT('',(-56.9777960240775,-81.7949165950883,19.6772168703845));
#44917=CARTESIAN_POINT('',(-56.9042068273237,-81.5494766841245,19.5999999999999));
#44918=CARTESIAN_POINT('Ctrl Pts',(-56.9777960279009,-81.7949165905344,
19.6772168782191));
#44919=CARTESIAN_POINT('Ctrl Pts',(-56.9774534269664,-81.7748789883664,
19.6657367803573));
#44920=CARTESIAN_POINT('Ctrl Pts',(-56.9758685115415,-81.7543927701849,
19.6551784083702));
#44921=CARTESIAN_POINT('Ctrl Pts',(-56.9671441435283,-81.6939687882869,
19.6278056262105));
#44922=CARTESIAN_POINT('Ctrl Pts',(-56.9562678019039,-81.6532801182632,
19.6140483572685));
#44923=CARTESIAN_POINT('Ctrl Pts',(-56.929299784212,-81.591434225957,19.6022201311171));
#44924=CARTESIAN_POINT('Ctrl Pts',(-56.9177055635009,-81.5698776231775,
19.5999999978021));
#44925=CARTESIAN_POINT('Ctrl Pts',(-56.904206824217,-81.5494766861803,19.6000000000003));
#44926=CARTESIAN_POINT('',(-56.8540093738152,-82.1084399539185,19.9814518777033));
#44927=CARTESIAN_POINT('Ctrl Pts',(-56.8540093738153,-82.1084399539186,
19.981451877705));
#44928=CARTESIAN_POINT('Ctrl Pts',(-56.8546684208551,-82.1078379696138,
19.9804667706938));
#44929=CARTESIAN_POINT('Ctrl Pts',(-56.8553252506811,-82.1072330983662,
19.9794819412701));
#44930=CARTESIAN_POINT('Ctrl Pts',(-56.885259036188,-82.0794420009762,19.9344611450319));
#44931=CARTESIAN_POINT('Ctrl Pts',(-56.9102018414315,-82.0463986825325,
19.8908548938768));
#44932=CARTESIAN_POINT('Ctrl Pts',(-56.9487731320942,-81.971873545886,19.8095675441362));
#44933=CARTESIAN_POINT('Ctrl Pts',(-56.9629285185929,-81.9303820655268,
19.7713797660207));
#44934=CARTESIAN_POINT('Ctrl Pts',(-56.9758152663889,-81.8565882282959,
19.7154512870322));
#44935=CARTESIAN_POINT('Ctrl Pts',(-56.9783326975642,-81.8263046345426,
19.6951999589232));
#44936=CARTESIAN_POINT('Ctrl Pts',(-56.9777960279009,-81.7949165905344,
19.6772168782191));
#44937=CARTESIAN_POINT('',(-56.3459906261847,-81.4915600460814,20.0185481222946));
#44938=CARTESIAN_POINT('Origin',(-56.6,-81.8,20.));
#44939=CARTESIAN_POINT('Ctrl Pts',(-56.904206824217,-81.5494766861803,19.6000000000003));
#44940=CARTESIAN_POINT('Ctrl Pts',(-56.8973970622138,-81.5391849453983,
19.6000000011092));
#44941=CARTESIAN_POINT('Ctrl Pts',(-56.8901026392551,-81.5291872963679,
19.6005647878238));
#44942=CARTESIAN_POINT('Ctrl Pts',(-56.8585917514376,-81.4901248771223,
19.6052302094125));
#44943=CARTESIAN_POINT('Ctrl Pts',(-56.8314688441805,-81.4653796121322,
19.6140191854886));
#44944=CARTESIAN_POINT('Ctrl Pts',(-56.7680758300491,-81.4230398883288,
19.642457690764));
#44945=CARTESIAN_POINT('Ctrl Pts',(-56.7324621427979,-81.4078826250911,
19.6628251782062));
#44946=CARTESIAN_POINT('Ctrl Pts',(-56.6455280686385,-81.3857136829775,
19.720036209981));
#44947=CARTESIAN_POINT('Ctrl Pts',(-56.5917170173975,-81.3846886026211,
19.7618502488057));
#44948=CARTESIAN_POINT('Ctrl Pts',(-56.4686735219491,-81.4084196738685,
19.8721932058865));
#44949=CARTESIAN_POINT('Ctrl Pts',(-56.4020317358757,-81.4415416401364,
19.9435530185242));
#44950=CARTESIAN_POINT('Ctrl Pts',(-56.3473237567345,-81.4903583244829,
20.016756128899));
#44951=CARTESIAN_POINT('Ctrl Pts',(-56.3466561735294,-81.4909580671593,
20.0176521239571));
#44952=CARTESIAN_POINT('Ctrl Pts',(-56.3459906261847,-81.4915600460814,
20.018548122295));
#44953=CARTESIAN_POINT('',(-58.4561395287659,-80.2714145057222,19.6));
#44954=CARTESIAN_POINT('',(-58.4561395287659,-80.2714145057222,19.6));
#44955=CARTESIAN_POINT('',(-58.4561395287659,-80.2714145057222,20.4));
#44956=CARTESIAN_POINT('Ctrl Pts',(-58.4561395287659,-80.2714145057222,
20.4));
#44957=CARTESIAN_POINT('Ctrl Pts',(-58.4549779405932,-80.2713020939635,
20.4));
#44958=CARTESIAN_POINT('Ctrl Pts',(-58.4538163849693,-80.2711893225306,
20.399997446394));
#44959=CARTESIAN_POINT('Ctrl Pts',(-58.3971341356222,-80.2656685650122,
20.3997479784273));
#44960=CARTESIAN_POINT('Ctrl Pts',(-58.3414898505613,-80.2594046889495,
20.3936592925489));
#44961=CARTESIAN_POINT('Ctrl Pts',(-58.2289948837902,-80.2452515766898,
20.3673459197356));
#44962=CARTESIAN_POINT('Ctrl Pts',(-58.1720125290647,-80.2372017088335,
20.3458022795996));
#44963=CARTESIAN_POINT('Ctrl Pts',(-58.0772658128868,-80.2227516349081,
20.2901288280491));
#44964=CARTESIAN_POINT('Ctrl Pts',(-58.0378581810609,-80.2163033472798,
20.258674501957));
#44965=CARTESIAN_POINT('Ctrl Pts',(-57.9781037597976,-80.2061585356058,
20.189514384551));
#44966=CARTESIAN_POINT('Ctrl Pts',(-57.9560095763437,-80.2022476217727,
20.1541222320853));
#44967=CARTESIAN_POINT('Ctrl Pts',(-57.9265724533894,-80.1969765246161,
20.0784874840272));
#44968=CARTESIAN_POINT('Ctrl Pts',(-57.9189967544966,-80.1955858364017,
20.0396265746691));
#44969=CARTESIAN_POINT('Ctrl Pts',(-57.9189967544966,-80.1955858364017,
19.9603734253309));
#44970=CARTESIAN_POINT('Ctrl Pts',(-57.9265724533894,-80.1969765246161,
19.9215125159728));
#44971=CARTESIAN_POINT('Ctrl Pts',(-57.9560095763437,-80.2022476217727,
19.8458777679147));
#44972=CARTESIAN_POINT('Ctrl Pts',(-57.9781037597976,-80.2061585356058,
19.810485615449));
#44973=CARTESIAN_POINT('Ctrl Pts',(-58.0378581810609,-80.2163033472798,
19.741325498043));
#44974=CARTESIAN_POINT('Ctrl Pts',(-58.0772658128868,-80.2227516349081,
19.7098711719509));
#44975=CARTESIAN_POINT('Ctrl Pts',(-58.1720125290647,-80.2372017088335,
19.6541977204004));
#44976=CARTESIAN_POINT('Ctrl Pts',(-58.2289948837902,-80.2452515766898,
19.6326540802644));
#44977=CARTESIAN_POINT('Ctrl Pts',(-58.3414898505845,-80.2594046889524,
19.6063407074457));
#44978=CARTESIAN_POINT('Ctrl Pts',(-58.3971341357726,-80.2656685650308,
19.6002520215721));
#44979=CARTESIAN_POINT('Ctrl Pts',(-58.4538163849616,-80.2711893225295,
19.600002553606));
#44980=CARTESIAN_POINT('Ctrl Pts',(-58.4549779406011,-80.2713020939643,
19.6));
#44981=CARTESIAN_POINT('Ctrl Pts',(-58.4561395287659,-80.2714145057222,
19.6));
#44982=CARTESIAN_POINT('Ctrl Pts',(-58.4561395287659,-80.2714145057222,
19.6));
#44983=CARTESIAN_POINT('Ctrl Pts',(-58.456027117008,-80.2725760938874,19.6));
#44984=CARTESIAN_POINT('Ctrl Pts',(-58.4559150644895,-80.2737377190986,
19.600002553606));
#44985=CARTESIAN_POINT('Ctrl Pts',(-58.4504644075707,-80.3304267522263,
19.6002520215721));
#44986=CARTESIAN_POINT('Ctrl Pts',(-58.4459421116762,-80.3862395774228,
19.6063407074461));
#44987=CARTESIAN_POINT('Ctrl Pts',(-58.4382613890477,-80.4993609045025,
19.6326540802644));
#44988=CARTESIAN_POINT('Ctrl Pts',(-58.4352353645325,-80.5568294376158,
19.6541977204004));
#44989=CARTESIAN_POINT('Ctrl Pts',(-58.4312493657365,-80.6525888062256,
19.7098711719509));
#44990=CARTESIAN_POINT('Ctrl Pts',(-58.4300214794505,-80.6925016381814,
19.741325498043));
#44991=CARTESIAN_POINT('Ctrl Pts',(-58.4285199726038,-80.753092508299,19.810485615449));
#44992=CARTESIAN_POINT('Ctrl Pts',(-58.4281216961571,-80.7755266244031,
19.8458777679147));
#44993=CARTESIAN_POINT('Ctrl Pts',(-58.4276503349443,-80.8054282379327,
19.9215125159728));
#44994=CARTESIAN_POINT('Ctrl Pts',(-58.4275625567855,-80.8131300248954,
19.9603734253309));
#44995=CARTESIAN_POINT('Ctrl Pts',(-58.4275625567855,-80.8131300248954,
20.0396265746691));
#44996=CARTESIAN_POINT('Ctrl Pts',(-58.4276503349443,-80.8054282379327,
20.0784874840272));
#44997=CARTESIAN_POINT('Ctrl Pts',(-58.4281216961571,-80.7755266244031,
20.1541222320853));
#44998=CARTESIAN_POINT('Ctrl Pts',(-58.4285199726038,-80.753092508299,20.189514384551));
#44999=CARTESIAN_POINT('Ctrl Pts',(-58.4300214794505,-80.6925016381814,
20.258674501957));
#45000=CARTESIAN_POINT('Ctrl Pts',(-58.4312493657365,-80.6525888062256,
20.2901288280491));
#45001=CARTESIAN_POINT('Ctrl Pts',(-58.4352353645325,-80.5568294376159,
20.3458022795996));
#45002=CARTESIAN_POINT('Ctrl Pts',(-58.4382613890477,-80.4993609045026,
20.3673459197356));
#45003=CARTESIAN_POINT('Ctrl Pts',(-58.4459421116747,-80.3862395774449,
20.3936592925487));
#45004=CARTESIAN_POINT('Ctrl Pts',(-58.4504644075606,-80.3304267523694,
20.3997479784273));
#45005=CARTESIAN_POINT('Ctrl Pts',(-58.4559150644899,-80.2737377190912,
20.399997446394));
#45006=CARTESIAN_POINT('Ctrl Pts',(-58.4560271170072,-80.272576093895,20.4));
#45007=CARTESIAN_POINT('Ctrl Pts',(-58.4561395287659,-80.2714145057222,
20.4));
#45008=CARTESIAN_POINT('Origin',(-56.6,-81.8,20.));
#45009=CARTESIAN_POINT('',(-56.6,-81.8,20.));
#45010=CARTESIAN_POINT('Origin',(-60.,-79.,20.));
#45011=CARTESIAN_POINT('',(-61.6,-79.,20.));
#45012=CARTESIAN_POINT('Origin',(-62.,-79.,20.));
#45013=CARTESIAN_POINT('Origin',(-60.,-79.,20.));
#45014=CARTESIAN_POINT('Origin',(-56.6,-81.8,20.));
#45015=CARTESIAN_POINT('Origin',(-56.6,-81.8,20.));
#45016=CARTESIAN_POINT('Ctrl Pts',(-56.998865393003,-81.8104071381607,19.971749517882));
#45017=CARTESIAN_POINT('Ctrl Pts',(-56.9761215679777,-81.8098137095668,
19.6504133876692));
#45018=CARTESIAN_POINT('Ctrl Pts',(-56.9306422269741,-81.702749946835,19.0272055496801));
#45019=CARTESIAN_POINT('Ctrl Pts',(-56.8393882333594,-81.0832286625891,
17.8952792144066));
#45020=CARTESIAN_POINT('Ctrl Pts',(-56.7246941823819,-79.659154025169,16.9983829421965));
#45021=CARTESIAN_POINT('Ctrl Pts',(-56.5861632252162,-77.6335534097869,
17.2233006398626));
#45022=CARTESIAN_POINT('Ctrl Pts',(-56.4467017882273,-76.1835978989143,
18.6719551219413));
#45023=CARTESIAN_POINT('Ctrl Pts',(-56.3063357852564,-75.9481362494154,
20.7219582178088));
#45024=CARTESIAN_POINT('Ctrl Pts',(-56.1650671343952,-77.0524010984881,
22.4820287706829));
#45025=CARTESIAN_POINT('Ctrl Pts',(-56.022913716882,-79.0240846877592,23.1743286974061));
#45026=CARTESIAN_POINT('Ctrl Pts',(-55.8798883483141,-81.0099417524087,
22.4819069016305));
#45027=CARTESIAN_POINT('Ctrl Pts',(-55.736009170698,-82.1371435389622,20.6919014148508));
#45028=CARTESIAN_POINT('Ctrl Pts',(-55.5912948188564,-81.9011989467447,
18.5773811983794));
#45029=CARTESIAN_POINT('Ctrl Pts',(-55.4457664679998,-80.3895075735084,
17.0631066199702));
#45030=CARTESIAN_POINT('Ctrl Pts',(-55.2994467925014,-78.2525981471427,
16.8201567755944));
#45031=CARTESIAN_POINT('Ctrl Pts',(-55.1523606723563,-76.4194586046196,
17.9695089930655));
#45032=CARTESIAN_POINT('Ctrl Pts',(-55.0291720750146,-75.8221765197523,
19.6778401981353));
#45033=CARTESIAN_POINT('Ctrl Pts',(-54.9302657004888,-76.0582767873485,
21.0517631272575));
#45034=CARTESIAN_POINT('Ctrl Pts',(-54.855911693957,-76.563774636797,21.9689095801494));
#45035=CARTESIAN_POINT('Ctrl Pts',(-54.7813873081152,-77.3470208623382,
22.6677199767267));
#45036=CARTESIAN_POINT('Ctrl Pts',(-54.6817995343713,-78.6425182874698,
23.2077559592215));
#45037=CARTESIAN_POINT('Ctrl Pts',(-54.5569085657542,-80.4660663250115,
23.0055515481889));
#45038=CARTESIAN_POINT('Ctrl Pts',(-54.4064224477222,-82.0323869212294,
21.4408137908159));
#45039=CARTESIAN_POINT('Ctrl Pts',(-54.2553538136249,-82.282138366727,19.2347828818201));
#45040=CARTESIAN_POINT('Ctrl Pts',(-54.1037383696759,-81.0976521492529,
17.3450468644423));
#45041=CARTESIAN_POINT('Ctrl Pts',(-53.9516134654316,-78.9865131673676,
16.6079479997978));
#45042=CARTESIAN_POINT('Ctrl Pts',(-53.799017300736,-76.8685737480114,17.3474746287888));
#45043=CARTESIAN_POINT('Ctrl Pts',(-53.6459896567803,-75.6706931696044,
19.2519276595415));
#45044=CARTESIAN_POINT('Ctrl Pts',(-53.4925710331048,-75.9223549441939,
21.4933728414198));
#45045=CARTESIAN_POINT('Ctrl Pts',(-53.3388026326536,-77.5204065688237,
23.0925152589881));
#45046=CARTESIAN_POINT('Ctrl Pts',(-53.1847265069516,-79.7714109640732,
23.3467986618763));
#45047=CARTESIAN_POINT('Ctrl Pts',(-53.03038548168,-81.6931375902356,22.1399790200489));
#45048=CARTESIAN_POINT('Ctrl Pts',(-52.875823002085,-82.4441600599385,19.9951637320667));
#45049=CARTESIAN_POINT('Ctrl Pts',(-52.7210833439104,-81.6931147568403,
17.847607587344));
#45050=CARTESIAN_POINT('Ctrl Pts',(-52.5662111784277,-79.7652472072559,
16.6359089985643));
#45051=CARTESIAN_POINT('Ctrl Pts',(-52.411251276088,-77.5012356580149,16.8908255535852));
#45052=CARTESIAN_POINT('Ctrl Pts',(-52.256248453475,-75.8897320482582,18.5022380823304));
#45053=CARTESIAN_POINT('Ctrl Pts',(-52.1012476567581,-75.6346189430596,
20.7668255842009));
#45054=CARTESIAN_POINT('Ctrl Pts',(-51.946293812071,-76.8468283649895,22.6957639240306));
#45055=CARTESIAN_POINT('Ctrl Pts',(-51.7914318627055,-78.9959989264195,
23.4475029895662));
#45056=CARTESIAN_POINT('Ctrl Pts',(-51.6367067716067,-81.143023685764,22.6958068198001));
#45057=CARTESIAN_POINT('Ctrl Pts',(-51.4821631962239,-82.3514430242135,
20.7716237421131));
#45058=CARTESIAN_POINT('Ctrl Pts',(-51.3278450629361,-82.0966921870304,
18.5171370441619));
#45059=CARTESIAN_POINT('Ctrl Pts',(-51.173795763927,-80.494660275846,16.9160818675009));
#45060=CARTESIAN_POINT('Ctrl Pts',(-51.0200579736735,-78.2481247248837,
16.6640082062395));
#45061=CARTESIAN_POINT('Ctrl Pts',(-50.8666737295509,-76.3395049302381,
17.8643638570452));
#45062=CARTESIAN_POINT('Ctrl Pts',(-50.713684168159,-75.5963279226902,19.9885708308413));
#45063=CARTESIAN_POINT('Ctrl Pts',(-50.561130291697,-76.3404917399077,22.103826159149));
#45064=CARTESIAN_POINT('Ctrl Pts',(-50.4090511127719,-78.2340315759714,
23.2925880511682));
#45065=CARTESIAN_POINT('Ctrl Pts',(-50.2574850343491,-80.4481760005255,
23.0417916058766));
#45066=CARTESIAN_POINT('Ctrl Pts',(-50.1064690255066,-82.01705159905,21.4708528285098));
#45067=CARTESIAN_POINT('Ctrl Pts',(-49.9560387185426,-82.2630418039423,
19.2728709293431));
#45068=CARTESIAN_POINT('Ctrl Pts',(-49.8062283566168,-81.0898252948096,
17.4088059239318));
#45069=CARTESIAN_POINT('Ctrl Pts',(-49.6570709537323,-79.019024315676,16.68592863221));
#45070=CARTESIAN_POINT('Ctrl Pts',(-49.5085980443133,-76.9595196408508,
17.4088734508976));
#45071=CARTESIAN_POINT('Ctrl Pts',(-49.3608396229039,-75.8040867405457,
19.24850872357));
#45072=CARTESIAN_POINT('Ctrl Pts',(-49.2138236838193,-76.0501675357259,
21.3978373023004));
#45073=CARTESIAN_POINT('Ctrl Pts',(-49.0675767596914,-77.5665861446786,
22.9130985070277));
#45074=CARTESIAN_POINT('Ctrl Pts',(-48.9059614999196,-79.9400679445208,
23.1852360004509));
#45075=CARTESIAN_POINT('Ctrl Pts',(-48.7614602181023,-81.6648094897616,
21.8082179781191));
#45076=CARTESIAN_POINT('Ctrl Pts',(-48.641745504212,-82.0326853928027,20.1333807208566));
#45077=CARTESIAN_POINT('Ctrl Pts',(-48.5622130344089,-81.8465385109611,
19.0326778475393));
#45078=CARTESIAN_POINT('Ctrl Pts',(-48.4670622745342,-81.1987085058851,
17.8562669615047));
#45079=CARTESIAN_POINT('Ctrl Pts',(-48.3486693000866,-79.7268341045547,
16.9318783271684));
#45080=CARTESIAN_POINT('Ctrl Pts',(-48.2074855512855,-77.6628755974866,
17.1663816685728));
#45081=CARTESIAN_POINT('Ctrl Pts',(-48.0672023078574,-76.206752176544,18.626431849987));
#45082=CARTESIAN_POINT('Ctrl Pts',(-47.927830219219,-75.9792981345661,20.6628912290644));
#45083=CARTESIAN_POINT('Ctrl Pts',(-47.7893778161085,-77.0643886294908,
22.3852565245146));
#45084=CARTESIAN_POINT('Ctrl Pts',(-47.6518515237459,-78.9735990241534,
23.0508787165266));
#45085=CARTESIAN_POINT('Ctrl Pts',(-47.5152556014389,-80.8684432520523,
22.3853788812134));
#45086=CARTESIAN_POINT('Ctrl Pts',(-47.3795921088708,-81.9276134623547,
20.6952758178572));
#45087=CARTESIAN_POINT('Ctrl Pts',(-47.2448609079158,-81.7034807862736,
18.7270982413631));
#45088=CARTESIAN_POINT('Ctrl Pts',(-47.1110596886693,-80.3107425715779,
17.3377494473466));
#45089=CARTESIAN_POINT('Ctrl Pts',(-46.9781840026693,-78.3691181398569,
17.1212491527646));
#45090=CARTESIAN_POINT('Ctrl Pts',(-46.8462272430603,-76.7274568500113,
18.1555514656259));
#45091=CARTESIAN_POINT('Ctrl Pts',(-46.7151806507337,-76.0932466642441,
19.9745644839421));
#45092=CARTESIAN_POINT('Ctrl Pts',(-46.5850332874596,-76.72689365866,21.7807592120224));
#45093=CARTESIAN_POINT('Ctrl Pts',(-46.4773155913697,-78.0692304834685,
22.6203028484064));
#45094=CARTESIAN_POINT('Ctrl Pts',(-46.3915770038462,-79.2743999206746,
22.6845333353118));
#45095=CARTESIAN_POINT('Ctrl Pts',(-46.306125933356,-80.4347163011863,22.3540877308873));
#45096=CARTESIAN_POINT('Ctrl Pts',(-46.2140165472685,-81.3855756228331,
21.3981264795911));
#45097=CARTESIAN_POINT('Ctrl Pts',(-46.0871761509613,-81.7920886092443,
19.6302877304961));
#45098=CARTESIAN_POINT('Ctrl Pts',(-45.9979124562317,-81.2080139528857,
18.4010685232934));
#45099=CARTESIAN_POINT('Ctrl Pts',(-45.931706785465,-80.4609863771443,17.8600692258404));
#45100=CARTESIAN_POINT('Ctrl Pts',(-45.8899254264441,-79.9656081265692,
17.5575209097683));
#45101=CARTESIAN_POINT('Ctrl Pts',(-45.8118000032237,-78.880763795498,17.2764338892227));
#45102=CARTESIAN_POINT('Ctrl Pts',(-45.6978306326569,-77.2975836321059,
17.8314065963964));
#45103=CARTESIAN_POINT('Ctrl Pts',(-45.5742396517875,-76.3354201599197,
19.3681907346036));
#45104=CARTESIAN_POINT('Ctrl Pts',(-45.437706343548,-76.5552758080846,21.3715656944865));
#45105=CARTESIAN_POINT('Ctrl Pts',(-45.3020562393531,-78.1821308742347,
22.6659223685449));
#45106=CARTESIAN_POINT('Ctrl Pts',(-45.1941987227426,-79.758928297719,22.475534026443));
#45107=CARTESIAN_POINT('Ctrl Pts',(-45.0866996199815,-81.0338356970261,
21.6807000396746));
#45108=CARTESIAN_POINT('Ctrl Pts',(-44.9662578644687,-81.8333475233177,
20.012518703382));
#45109=CARTESIAN_POINT('Ctrl Pts',(-44.8243750512167,-80.8834891862673,
18.0522457056093));
#45110=CARTESIAN_POINT('Ctrl Pts',(-44.7007996247099,-79.204627825654,17.4066536628875));
#45111=CARTESIAN_POINT('Ctrl Pts',(-44.5952423985192,-77.7129206082217,
17.7439551046314));
#45112=CARTESIAN_POINT('Ctrl Pts',(-44.4900223228441,-76.6730225954323,
18.8674759604783));
#45113=CARTESIAN_POINT('Ctrl Pts',(-44.3851107070103,-76.4459242852341,
20.3731595407077));
#45114=CARTESIAN_POINT('Ctrl Pts',(-44.280478717402,-77.1066399045476,21.7436998539951));
#45115=CARTESIAN_POINT('Ctrl Pts',(-44.1847949217249,-78.3107241896412,
22.4370140832109));
#45116=CARTESIAN_POINT('Ctrl Pts',(-44.0979705969536,-79.5480359338008,
22.4357585099148));
#45117=CARTESIAN_POINT('Ctrl Pts',(-44.0199391969229,-80.5493767638303,
21.9538965049427));
#45118=CARTESIAN_POINT('Ctrl Pts',(-43.9549950707645,-81.1260138276735,
21.230332507434));
#45119=CARTESIAN_POINT('Ctrl Pts',(-43.9030819779796,-81.3650788043183,
20.5453498510557));
#45120=CARTESIAN_POINT('Ctrl Pts',(-43.8511952002441,-81.4469675514213,
19.8246440252031));
#45121=CARTESIAN_POINT('Ctrl Pts',(-43.786381545381,-81.2412693616971,18.9250357363984));
#45122=CARTESIAN_POINT('Ctrl Pts',(-43.7086639057346,-80.5513181773471,
18.058939887935));
#45123=CARTESIAN_POINT('Ctrl Pts',(-43.6309915965552,-79.554575354439,17.5802369898606));
#45124=CARTESIAN_POINT('Ctrl Pts',(-43.5404114400028,-78.2638755524742,
17.5781557379155));
#45125=CARTESIAN_POINT('Ctrl Pts',(-43.4369226415031,-76.9748964799918,
18.3837836136963));
#45126=CARTESIAN_POINT('Ctrl Pts',(-43.3204955018513,-76.409902299744,20.0015897439));
#45127=CARTESIAN_POINT('Ctrl Pts',(-43.2040204721867,-76.9752002181154,
21.6172377254714));
#45128=CARTESIAN_POINT('Ctrl Pts',(-43.0874525410452,-78.4262949071933,
22.5297854402615));
#45129=CARTESIAN_POINT('Ctrl Pts',(-42.9707470684933,-80.1313821068561,
22.3379694555197));
#45130=CARTESIAN_POINT('Ctrl Pts',(-42.8538596468785,-81.3469559099921,
21.1232848086745));
#45131=CARTESIAN_POINT('Ctrl Pts',(-42.7367469025614,-81.5402924255104,
19.4123612569526));
#45132=CARTESIAN_POINT('Ctrl Pts',(-42.6193646471204,-80.6227499332965,
17.950746393619));
#45133=CARTESIAN_POINT('Ctrl Pts',(-42.5016723128577,-78.9894841983059,
17.3785603509998));
#45134=CARTESIAN_POINT('Ctrl Pts',(-42.3836228189166,-77.3512439815465,
17.9509054109146));
#45135=CARTESIAN_POINT('Ctrl Pts',(-42.2651858183516,-76.4228942839963,
19.4252147114051));
#45136=CARTESIAN_POINT('Ctrl Pts',(-42.1462969423314,-76.6193425219703,
21.1617531840419));
#45137=CARTESIAN_POINT('Ctrl Pts',(-42.0269611323496,-77.8579790787978,
22.4041645790426));
#45138=CARTESIAN_POINT('Ctrl Pts',(-41.9070542715169,-79.6104428558897,
22.601547445429));
#45139=CARTESIAN_POINT('Ctrl Pts',(-41.8067886921112,-80.8577927602762,
21.8204122976217));
#45140=CARTESIAN_POINT('Ctrl Pts',(-41.7260879027667,-81.4058116777841,
20.8193752889488));
#45141=CARTESIAN_POINT('Ctrl Pts',(-41.6858137213157,-81.5009183081234,
20.2675948162325));
#45142=CARTESIAN_POINT('Ctrl Pts',(-41.6655045384048,-81.5014482121737,
19.980656523783));
#45143=CARTESIAN_POINT('Ctrl Pts',(-57.0019869965663,-81.6907681353096,
19.971749517882));
#45144=CARTESIAN_POINT('Ctrl Pts',(-56.9801545695107,-81.6901984867797,
19.663290073818));
#45145=CARTESIAN_POINT('Ctrl Pts',(-56.9366454549946,-81.5877436991947,
19.0670363519488));
#45146=CARTESIAN_POINT('Ctrl Pts',(-56.8491846045637,-80.9941573968246,
17.9820163561888));
#45147=CARTESIAN_POINT('Ctrl Pts',(-56.7393118494271,-79.6295959629488,
17.1227663162549));
#45148=CARTESIAN_POINT('Ctrl Pts',(-56.6064781904435,-77.6872334681487,
17.3380508628845));
#45149=CARTESIAN_POINT('Ctrl Pts',(-56.4726828633942,-76.2958461360222,
18.7279994719948));
#45150=CARTESIAN_POINT('Ctrl Pts',(-56.3379160681303,-76.0694886906288,
20.6963932339323));
#45151=CARTESIAN_POINT('Ctrl Pts',(-56.2021929256842,-77.1304743295524,
22.3880320262854));
#45152=CARTESIAN_POINT('Ctrl Pts',(-56.0654858506924,-79.0269074027327,
23.0542475046959));
#45153=CARTESIAN_POINT('Ctrl Pts',(-55.9278104502865,-80.9390721595663,
22.3879092034606));
#45154=CARTESIAN_POINT('Ctrl Pts',(-55.7891657233314,-82.0258490619999,
20.6628380569866));
#45155=CARTESIAN_POINT('Ctrl Pts',(-55.6495621609665,-81.7986045584916,
18.6224539012947));
#45156=CARTESIAN_POINT('Ctrl Pts',(-55.5090063278671,-80.3385390793215,
17.15925969508));
#45157=CARTESIAN_POINT('Ctrl Pts',(-55.367513994765,-78.2716513700982,16.9237976938686));
#45158=CARTESIAN_POINT('Ctrl Pts',(-55.2250902663515,-76.4959591428919,
18.0365569888073));
#45159=CARTESIAN_POINT('Ctrl Pts',(-55.1056572247686,-75.9163181618903,
19.6932190528411));
#45160=CARTESIAN_POINT('Ctrl Pts',(-55.0096417192807,-76.1454620591887,
21.0271736310102));
#45161=CARTESIAN_POINT('Ctrl Pts',(-54.9374115962142,-76.6365391415173,
21.918279169925));
#45162=CARTESIAN_POINT('Ctrl Pts',(-54.8649633201778,-77.398040791451,22.5977776331588));
#45163=CARTESIAN_POINT('Ctrl Pts',(-54.7680757073581,-78.6585216738225,
23.1233216086256));
#45164=CARTESIAN_POINT('Ctrl Pts',(-54.6464650009296,-80.4348314338745,
22.9268255090038));
#45165=CARTESIAN_POINT('Ctrl Pts',(-54.4996934767181,-81.9633416794487,
21.4007041190596));
#45166=CARTESIAN_POINT('Ctrl Pts',(-54.3521194914096,-82.207945805232,19.2451779007863));
#45167=CARTESIAN_POINT('Ctrl Pts',(-54.2037864512958,-81.0491986386383,
17.3953506314354));
#45168=CARTESIAN_POINT('Ctrl Pts',(-54.0546726002324,-78.9797161272989,
16.6721627753971));
#45169=CARTESIAN_POINT('Ctrl Pts',(-53.9048744917015,-76.8997385794412,
17.3977515494516));
#45170=CARTESIAN_POINT('Ctrl Pts',(-53.7543943945856,-75.7208910787165,
19.2707235463476));
#45171=CARTESIAN_POINT('Ctrl Pts',(-53.6032700366971,-75.9682122953648,
21.4793965483087));
#45172=CARTESIAN_POINT('Ctrl Pts',(-53.4515364940605,-77.5451237531408,
23.0583259880909));
#45173=CARTESIAN_POINT('Ctrl Pts',(-53.2992315669793,-79.7708514113732,
23.3104301280262));
#45174=CARTESIAN_POINT('Ctrl Pts',(-53.1463938538412,-81.674796438284,22.1155785760537));
#45175=CARTESIAN_POINT('Ctrl Pts',(-52.9930634292223,-82.4207031937924,
19.9874447955775));
#45176=CARTESIAN_POINT('Ctrl Pts',(-52.8392816877573,-81.674734243082,17.8523154647485));
#45177=CARTESIAN_POINT('Ctrl Pts',(-52.685091115623,-79.7551482890924,16.6450035815774));
#45178=CARTESIAN_POINT('Ctrl Pts',(-52.5305349248319,-77.4962905952853,
16.8986406907687));
#45179=CARTESIAN_POINT('Ctrl Pts',(-52.3756570363291,-75.8851236735628,
18.5087336570864));
#45180=CARTESIAN_POINT('Ctrl Pts',(-52.2205021178324,-75.6289937996702,
20.7761504419683));
#45181=CARTESIAN_POINT('Ctrl Pts',(-52.0651155111308,-76.8443509963939,
22.7113962588161));
#45182=CARTESIAN_POINT('Ctrl Pts',(-51.9095431202422,-79.0037626673798,
23.4674453589518));
#45183=CARTESIAN_POINT('Ctrl Pts',(-51.7538317605233,-81.1653007981464,
22.7113908580931));
#45184=CARTESIAN_POINT('Ctrl Pts',(-51.5980280916369,-82.3844800346085,
20.7713497617126));
#45185=CARTESIAN_POINT('Ctrl Pts',(-51.4421798125795,-82.1278008744938,
18.4938138332471));
#45186=CARTESIAN_POINT('Ctrl Pts',(-51.2863321673339,-80.5071214327334,
16.8731800143954));
#45187=CARTESIAN_POINT('Ctrl Pts',(-51.130536019338,-78.2299651325731,16.6170046250107));
#45188=CARTESIAN_POINT('Ctrl Pts',(-50.9748294395751,-76.2916779025706,
17.8352675022703));
#45189=CARTESIAN_POINT('Ctrl Pts',(-50.8192788139203,-75.535222425711,19.9954618233132));
#45190=CARTESIAN_POINT('Ctrl Pts',(-50.6638867930748,-76.2927555227092,
22.1505393874449));
#45191=CARTESIAN_POINT('Ctrl Pts',(-50.5087514726537,-78.2244666356574,
23.3639881816775));
#45192=CARTESIAN_POINT('Ctrl Pts',(-50.3538945398054,-80.4872358031265,
23.1082751603607));
#45193=CARTESIAN_POINT('Ctrl Pts',(-50.1993628432606,-82.0933694651835,
21.5008310722846));
#45194=CARTESIAN_POINT('Ctrl Pts',(-50.0451997389494,-82.3460604904031,
19.2479176258722));
#45195=CARTESIAN_POINT('Ctrl Pts',(-49.8914483697448,-81.1422016319754,
17.3341629878747));
#45196=CARTESIAN_POINT('Ctrl Pts',(-49.7381512549702,-79.0137037469387,
16.5905910347466));
#45197=CARTESIAN_POINT('Ctrl Pts',(-49.5853491463611,-76.8936172217032,
17.3342716101559));
#45198=CARTESIAN_POINT('Ctrl Pts',(-49.4330838300899,-75.7023254250077,
19.23006834526));
#45199=CARTESIAN_POINT('Ctrl Pts',(-49.2813906500908,-75.9558173014907,
21.4481635243258));
#45200=CARTESIAN_POINT('Ctrl Pts',(-49.1303147410793,-77.5222584825662,
23.0139808902264));
#45201=CARTESIAN_POINT('Ctrl Pts',(-48.9631599505202,-79.9772604688309,
23.2959931188457));
#45202=CARTESIAN_POINT('Ctrl Pts',(-48.8135053288752,-81.7639158613361,
21.8703489536029));
#45203=CARTESIAN_POINT('Ctrl Pts',(-48.6894028260435,-82.1454765472973,
20.1340332249349));
#45204=CARTESIAN_POINT('Ctrl Pts',(-48.606909800781,-81.9524122938921,18.9923151182377));
#45205=CARTESIAN_POINT('Ctrl Pts',(-48.508170467145,-81.2801964984991,17.7714890537002));
#45206=CARTESIAN_POINT('Ctrl Pts',(-48.3852366463024,-79.7519113147864,
16.811404479291));
#45207=CARTESIAN_POINT('Ctrl Pts',(-48.2385155735682,-77.6069227684042,
17.0548447507493));
#45208=CARTESIAN_POINT('Ctrl Pts',(-48.0926237391039,-76.0923857542406,
18.5731419517954));
#45209=CARTESIAN_POINT('Ctrl Pts',(-47.947583021408,-75.855478330155,20.6924131824904));
#45210=CARTESIAN_POINT('Ctrl Pts',(-47.8034159184779,-76.9851960001735,
22.4859469609739));
#45211=CARTESIAN_POINT('Ctrl Pts',(-47.6601418264662,-78.9740985729673,
23.1795079552557));
#45212=CARTESIAN_POINT('Ctrl Pts',(-47.5177785879326,-80.9488982642021,
22.4860500718809));
#45213=CARTESIAN_POINT('Ctrl Pts',(-47.3763417219138,-82.0531474374999,
20.7241762413299));
#45214=CARTESIAN_POINT('Ctrl Pts',(-47.235844434292,-81.8194952609905,18.6719275218613));
#45215=CARTESIAN_POINT('Ctrl Pts',(-47.0962979916432,-80.3671156551725,
17.2230535256656));
#45216=CARTESIAN_POINT('Ctrl Pts',(-46.9577106913804,-78.3422825162418,
16.9972911628132));
#45217=CARTESIAN_POINT('Ctrl Pts',(-46.8200902726817,-76.6304302822888,
18.075883028566));
#45218=CARTESIAN_POINT('Ctrl Pts',(-46.6834384403178,-75.9693039379864,
19.9724034084133));
#45219=CARTESIAN_POINT('Ctrl Pts',(-46.5477630195146,-76.6298878847089,
21.8549661590069));
#45220=CARTESIAN_POINT('Ctrl Pts',(-46.4355022701039,-78.0285744887402,
22.7295728438287));
#45221=CARTESIAN_POINT('Ctrl Pts',(-46.3461948648046,-79.2837766671998,
22.7964336666031));
#45222=CARTESIAN_POINT('Ctrl Pts',(-46.2572098972965,-80.491947115071,22.4523137524949));
#45223=CARTESIAN_POINT('Ctrl Pts',(-46.1613273153243,-81.4814786400232,
21.4572593980856));
#45224=CARTESIAN_POINT('Ctrl Pts',(-46.029379168661,-81.9042028287135,19.6183514631787));
#45225=CARTESIAN_POINT('Ctrl Pts',(-45.9365841068927,-81.2968358878326,
18.3408380995742));
#45226=CARTESIAN_POINT('Ctrl Pts',(-45.8678105576775,-80.5209218669219,
17.7789311757114));
#45227=CARTESIAN_POINT('Ctrl Pts',(-45.8244172040792,-80.0064507564458,
17.4647228951126));
#45228=CARTESIAN_POINT('Ctrl Pts',(-45.7433029268672,-78.8802013286524,
17.1730202319442));
#45229=CARTESIAN_POINT('Ctrl Pts',(-45.625023158468,-77.238153925619,17.749002446988));
#45230=CARTESIAN_POINT('Ctrl Pts',(-45.4969734702573,-76.2416278070243,
19.3413279722522));
#45231=CARTESIAN_POINT('Ctrl Pts',(-45.3556138735636,-76.4696516892768,
21.4144303969982));
#45232=CARTESIAN_POINT('Ctrl Pts',(-45.2154337533091,-78.1509909287844,
22.7510113308197));
#45233=CARTESIAN_POINT('Ctrl Pts',(-45.1041545433855,-79.77719143669,22.5542299247681));
#45234=CARTESIAN_POINT('Ctrl Pts',(-44.9933799101428,-81.0907403963799,
21.7352269105764));
#45235=CARTESIAN_POINT('Ctrl Pts',(-44.8694102564831,-81.9125541069559,
20.0183583220098));
#45236=CARTESIAN_POINT('Ctrl Pts',(-44.7237191663694,-80.9363612867671,
18.0064421148482));
#45237=CARTESIAN_POINT('Ctrl Pts',(-44.5970462847396,-79.2162221332394,
17.3455095591394));
#45238=CARTESIAN_POINT('Ctrl Pts',(-44.4890652688093,-77.6906315220753,
17.6908462673951));
#45239=CARTESIAN_POINT('Ctrl Pts',(-44.3815708076311,-76.6292107816859,
18.8382383324711));
#45240=CARTESIAN_POINT('Ctrl Pts',(-44.2746354502652,-76.3982162105429,
20.3727555213266));
#45241=CARTESIAN_POINT('Ctrl Pts',(-44.1681351294007,-77.0707409099873,
21.7667200651887));
#45242=CARTESIAN_POINT('Ctrl Pts',(-44.0709442472466,-78.2934511464485,
22.4702571756528));
#45243=CARTESIAN_POINT('Ctrl Pts',(-43.982911287045,-79.5475054890082,22.4687580004392));
#45244=CARTESIAN_POINT('Ctrl Pts',(-43.9039153234828,-80.560817283634,21.9809254218161));
#45245=CARTESIAN_POINT('Ctrl Pts',(-43.8382577690521,-81.1433928581717,
21.2496464767121));
#45246=CARTESIAN_POINT('Ctrl Pts',(-43.7858541652558,-81.384655107603,20.5582833734644));
#45247=CARTESIAN_POINT('Ctrl Pts',(-43.7335111620554,-81.46720801557,19.8314057389319));
#45248=CARTESIAN_POINT('Ctrl Pts',(-43.668205947399,-81.2598502135044,18.9251965418744));
#45249=CARTESIAN_POINT('Ctrl Pts',(-43.5900171832591,-80.5657229312084,
18.0541956163639));
#45250=CARTESIAN_POINT('Ctrl Pts',(-43.5119949360051,-79.5647038944138,
17.5736303297245));
#45251=CARTESIAN_POINT('Ctrl Pts',(-43.4211637692904,-78.2706023916298,
17.5717877335082));
#45252=CARTESIAN_POINT('Ctrl Pts',(-43.3175670029884,-76.9810666086263,
18.3784566755502));
#45253=CARTESIAN_POINT('Ctrl Pts',(-43.2012797062853,-76.4177083926015,
19.9937013177312));
#45254=CARTESIAN_POINT('Ctrl Pts',(-43.0852342760176,-76.9813003440223,
21.602448212408));
#45255=CARTESIAN_POINT('Ctrl Pts',(-42.9693708727529,-78.4233112003797,
22.5084979989942));
#45256=CARTESIAN_POINT('Ctrl Pts',(-42.8536484379065,-80.1132146170046,
22.3177218418165));
#45257=CARTESIAN_POINT('Ctrl Pts',(-42.7380174315994,-81.3147326529136,
21.1161627237155));
#45258=CARTESIAN_POINT('Ctrl Pts',(-42.622431553402,-81.5048285111816,19.4282173657));
#45259=CARTESIAN_POINT('Ctrl Pts',(-42.5068436055692,-80.6011664819877,
17.9899070717688));
#45260=CARTESIAN_POINT('Ctrl Pts',(-42.3912050559913,-78.9969340372162,
17.4285740592569));
#45261=CARTESIAN_POINT('Ctrl Pts',(-42.275471116222,-77.3917022239558,17.9900550824597));
#45262=CARTESIAN_POINT('Ctrl Pts',(-42.1595879125518,-76.484399288327,19.4322227612078));
#45263=CARTESIAN_POINT('Ctrl Pts',(-42.0435230131546,-76.6767317876591,
21.126904131581));
#45264=CARTESIAN_POINT('Ctrl Pts',(-41.9272646554307,-77.8836619438754,
22.3367466196967));
#45265=CARTESIAN_POINT('Ctrl Pts',(-41.8106510944935,-79.5876128552717,
22.5280006580125));
#45266=CARTESIAN_POINT('Ctrl Pts',(-41.7133341547954,-80.7980091014391,
21.7698238788751));
#45267=CARTESIAN_POINT('Ctrl Pts',(-41.6350706349544,-81.3292252397651,
20.7991118311558));
#45268=CARTESIAN_POINT('Ctrl Pts',(-41.596096236417,-81.4212850362297,20.2652300023777));
#45269=CARTESIAN_POINT('Ctrl Pts',(-41.5763904523584,-81.4217991964907,
19.9868168306642));
#45270=CARTESIAN_POINT('Ctrl Pts',(-56.8938806655278,-81.449218908126,19.9798472493564));
#45271=CARTESIAN_POINT('Ctrl Pts',(-56.8739034306165,-81.4486976650013,
19.6975988873676));
#45272=CARTESIAN_POINT('Ctrl Pts',(-56.834388516913,-81.3555481289854,19.1561130599078));
#45273=CARTESIAN_POINT('Ctrl Pts',(-56.754710817907,-80.81511613009,18.1675547779568));
#45274=CARTESIAN_POINT('Ctrl Pts',(-56.6548967662929,-79.5747336327388,
17.3876045355145));
#45275=CARTESIAN_POINT('Ctrl Pts',(-56.5342263208108,-77.8106208453556,
17.5830023129393));
#45276=CARTESIAN_POINT('Ctrl Pts',(-56.4128097095029,-76.5479937245359,
18.8448683450199));
#45277=CARTESIAN_POINT('Ctrl Pts',(-56.2905391787879,-76.3427409187718,
20.6305435185828));
#45278=CARTESIAN_POINT('Ctrl Pts',(-56.1674316415267,-77.3051540077992,
22.1650049810762));
#45279=CARTESIAN_POINT('Ctrl Pts',(-56.0434183804932,-79.0253682692881,
22.7693699258002));
#45280=CARTESIAN_POINT('Ctrl Pts',(-55.9184902021531,-80.76041430407,22.1649257307675));
#45281=CARTESIAN_POINT('Ctrl Pts',(-55.7926139794339,-81.7471752563372,
20.5989990927192));
#45282=CARTESIAN_POINT('Ctrl Pts',(-55.665770759842,-81.5409899392144,18.7453244956607));
#45283=CARTESIAN_POINT('Ctrl Pts',(-55.5379380211753,-80.2134922663367,
17.4145335706771));
#45284=CARTESIAN_POINT('Ctrl Pts',(-55.4090994105114,-78.3317895941842,
17.199794799748));
#45285=CARTESIAN_POINT('Ctrl Pts',(-55.2792362147139,-76.7126809740671,
18.2138816022247));
#45286=CARTESIAN_POINT('Ctrl Pts',(-55.1701567495123,-76.1829937999486,
19.7264829493925));
#45287=CARTESIAN_POINT('Ctrl Pts',(-55.0823625588476,-76.3924030320099,
20.9461543340251));
#45288=CARTESIAN_POINT('Ctrl Pts',(-55.0162545425101,-76.8417463674681,
21.7616744562217));
#45289=CARTESIAN_POINT('Ctrl Pts',(-54.9498823613353,-77.539261345362,22.3841725264662));
#45290=CARTESIAN_POINT('Ctrl Pts',(-54.8610323667072,-78.6949935525488,
22.8661593057298));
#45291=CARTESIAN_POINT('Ctrl Pts',(-54.7493114127749,-80.3264380739757,
22.6862663557752));
#45292=CARTESIAN_POINT('Ctrl Pts',(-54.6141770440791,-81.7339723863005,
21.282048149325));
#45293=CARTESIAN_POINT('Ctrl Pts',(-54.4779752619141,-81.9605162195905,
19.2931923197602));
#45294=CARTESIAN_POINT('Ctrl Pts',(-54.3407073175252,-80.8893439419391,
17.5814556098495));
#45295=CARTESIAN_POINT('Ctrl Pts',(-54.2023736536333,-78.9700251318391,
16.9097214459956));
#45296=CARTESIAN_POINT('Ctrl Pts',(-54.0629841015741,-77.0348423863016,
17.5837533254939));
#45297=CARTESIAN_POINT('Ctrl Pts',(-53.9225461836219,-75.9341039807705,
19.3306551916095));
#45298=CARTESIAN_POINT('Ctrl Pts',(-53.7810707929938,-76.1644712152157,
21.397800765737));
#45299=CARTESIAN_POINT('Ctrl Pts',(-53.6385714735097,-77.6441441078143,
22.8809897524166));
#45300=CARTESIAN_POINT('Ctrl Pts',(-53.4950639676803,-79.740509330956,23.1196407622332));
#45301=CARTESIAN_POINT('Ctrl Pts',(-53.3505664751887,-81.5406299938883,
21.9913998749732));
#45302=CARTESIAN_POINT('Ctrl Pts',(-53.2050994521972,-82.2492481514294,
19.9734896793798));
#45303=CARTESIAN_POINT('Ctrl Pts',(-53.0586858006082,-81.540488114762,17.9409077358488));
#45304=CARTESIAN_POINT('Ctrl Pts',(-52.9113506491857,-79.7075778778228,
16.7865308434111));
#45305=CARTESIAN_POINT('Ctrl Pts',(-52.7631211786402,-77.5417692000642,
17.0283429800463));
#45306=CARTESIAN_POINT('Ctrl Pts',(-52.6140265379999,-75.9903067164397,
18.5767943577803));
#45307=CARTESIAN_POINT('Ctrl Pts',(-52.4640979081661,-75.7414723756217,
20.7669193990113));
#45308=CARTESIAN_POINT('Ctrl Pts',(-52.3133683735114,-76.9187653495364,
22.6442841363996));
#45309=CARTESIAN_POINT('Ctrl Pts',(-52.1618730139186,-79.0203650036271,
23.381653056446));
#45310=CARTESIAN_POINT('Ctrl Pts',(-52.0096487974204,-81.1332438312709,
22.6441978412598));
#45311=CARTESIAN_POINT('Ctrl Pts',(-51.8567346701536,-82.3306671274323,
20.7416040561834));
#45312=CARTESIAN_POINT('Ctrl Pts',(-51.703170408764,-82.0793436505482,18.4980732665105));
#45313=CARTESIAN_POINT('Ctrl Pts',(-51.548998435844,-80.4777166500322,16.8943328305896));
#45314=CARTESIAN_POINT('Ctrl Pts',(-51.3942599140222,-78.2170100179401,
16.6384668010765));
#45315=CARTESIAN_POINT('Ctrl Pts',(-51.2390031714738,-76.2840963807832,
17.8515302441033));
#45316=CARTESIAN_POINT('Ctrl Pts',(-51.0832647073186,-75.5255777659518,
20.0128901467821));
#45317=CARTESIAN_POINT('Ctrl Pts',(-50.9271121506165,-76.2852475855935,
22.1787168558586));
#45318=CARTESIAN_POINT('Ctrl Pts',(-50.77056825008,-78.2330104312193,23.4040514047276));
#45319=CARTESIAN_POINT('Ctrl Pts',(-50.6136938502426,-80.524688911548,23.1466211054636));
#45320=CARTESIAN_POINT('Ctrl Pts',(-50.4565368618462,-82.1586749532148,
21.5134827334387));
#45321=CARTESIAN_POINT('Ctrl Pts',(-50.2991475798848,-82.4180954974584,
19.2143218707712));
#45322=CARTESIAN_POINT('Ctrl Pts',(-50.1415762807599,-81.1860035174916,
17.2528324014937));
#45323=CARTESIAN_POINT('Ctrl Pts',(-49.9838738197086,-78.9975177621074,
16.486714827865));
#45324=CARTESIAN_POINT('Ctrl Pts',(-49.8260923486205,-76.8085272901581,
17.253030288183));
#45325=CARTESIAN_POINT('Ctrl Pts',(-49.6682820790183,-75.5730195227687,
19.216469125723));
#45326=CARTESIAN_POINT('Ctrl Pts',(-49.5104978361797,-75.8352207050452,
21.5232288242989));
#45327=CARTESIAN_POINT('Ctrl Pts',(-49.3527832636632,-77.4690060053744,
23.1581845435753));
#45328=CARTESIAN_POINT('Ctrl Pts',(-49.1776977284958,-80.0397589837405,
23.4552962194859));
#45329=CARTESIAN_POINT('Ctrl Pts',(-49.0203423715508,-81.9195835809123,
21.9580643192054));
#45330=CARTESIAN_POINT('Ctrl Pts',(-48.8894100336456,-82.3227846164501,
20.1263666907));
#45331=CARTESIAN_POINT('Ctrl Pts',(-48.8022107925218,-82.1188190468183,
18.9196473910859));
#45332=CARTESIAN_POINT('Ctrl Pts',(-48.6976764064176,-81.4074504860157,
17.6271971643817));
#45333=CARTESIAN_POINT('Ctrl Pts',(-48.5671956740568,-79.7862474292538,
16.6075671275254));
#45334=CARTESIAN_POINT('Ctrl Pts',(-48.4110057336366,-77.5030478338066,
16.86546764075));
#45335=CARTESIAN_POINT('Ctrl Pts',(-48.2552376689688,-75.8854225102068,
18.4854612464013));
#45336=CARTESIAN_POINT('Ctrl Pts',(-48.0999434436653,-75.6307100332678,
20.7541124518367));
#45337=CARTESIAN_POINT('Ctrl Pts',(-47.9451661206175,-76.8425294742725,
22.6799565976964));
#45338=CARTESIAN_POINT('Ctrl Pts',(-47.7909512523896,-78.9827633245282,
23.4273301176066));
#45339=CARTESIAN_POINT('Ctrl Pts',(-47.6373416660037,-81.1136922956471,
22.6800260682271));
#45340=CARTESIAN_POINT('Ctrl Pts',(-47.4843795207015,-82.3085819854583,
20.7751611932815));
#45341=CARTESIAN_POINT('Ctrl Pts',(-47.3321048269705,-82.0561553777343,
18.5508802879414));
#45342=CARTESIAN_POINT('Ctrl Pts',(-47.1805562855874,-80.4794196831413,
16.9768948333079));
#45343=CARTESIAN_POINT('Ctrl Pts',(-47.029770256272,-78.2764296948284,16.7305760045727));
#45344=CARTESIAN_POINT('Ctrl Pts',(-46.8797825692249,-76.4103691501619,
17.9055895262826));
#45345=CARTESIAN_POINT('Ctrl Pts',(-46.7306246774405,-75.6881729894422,
19.9755811261626));
#45346=CARTESIAN_POINT('Ctrl Pts',(-46.5823318642751,-76.4097535506971,
22.0334906631283));
#45347=CARTESIAN_POINT('Ctrl Pts',(-46.4594923341318,-77.9402056822882,
22.9909089774758));
#45348=CARTESIAN_POINT('Ctrl Pts',(-46.3616909254776,-79.314859900965,23.0641907370176));
#45349=CARTESIAN_POINT('Ctrl Pts',(-46.2641995052703,-80.6385976410735,
22.6872274238976));
#45350=CARTESIAN_POINT('Ctrl Pts',(-46.1590932556085,-81.7235437390656,
21.596478187795));
#45351=CARTESIAN_POINT('Ctrl Pts',(-46.014372674255,-82.1873157419008,19.5794806256373));
#45352=CARTESIAN_POINT('Ctrl Pts',(-45.9125554805191,-81.5209695292361,
18.1775553804498));
#45353=CARTESIAN_POINT('Ctrl Pts',(-45.8370809471352,-80.6693842884602,
17.5608521824556));
#45354=CARTESIAN_POINT('Ctrl Pts',(-45.7894563496702,-80.104733110141,17.2159936869747));
#45355=CARTESIAN_POINT('Ctrl Pts',(-45.7004335623306,-78.8685673337143,
16.8958075847323));
#45356=CARTESIAN_POINT('Ctrl Pts',(-45.5706717427821,-77.0663809967464,
17.5279735658841));
#45357=CARTESIAN_POINT('Ctrl Pts',(-45.430169690343,-75.9729867562349,19.2752779146581));
#45358=CARTESIAN_POINT('Ctrl Pts',(-45.2752021281552,-76.2233068312271,
21.5489130349393));
#45359=CARTESIAN_POINT('Ctrl Pts',(-45.1216158714685,-78.0661371879358,
23.0131504465605));
#45360=CARTESIAN_POINT('Ctrl Pts',(-44.9998479620023,-79.8459952382941,
22.7973970035329));
#45361=CARTESIAN_POINT('Ctrl Pts',(-44.8787164843353,-81.2825728142914,
21.9016562184237));
#45362=CARTESIAN_POINT('Ctrl Pts',(-44.7433295404188,-82.1794770296741,
20.0257518112265));
#45363=CARTESIAN_POINT('Ctrl Pts',(-44.5845594999856,-81.1142670786869,
17.8332659205346));
#45364=CARTESIAN_POINT('Ctrl Pts',(-44.4468550226416,-79.2432620245245,
17.1150869676367));
#45365=CARTESIAN_POINT('Ctrl Pts',(-44.3296591566119,-77.5872330042658,
17.4904086854693));
#45366=CARTESIAN_POINT('Ctrl Pts',(-44.2132882540016,-76.4379280034599,
18.733713586435));
#45367=CARTESIAN_POINT('Ctrl Pts',(-44.0977385940157,-76.1888336362038,
20.3922467063092));
#45368=CARTESIAN_POINT('Ctrl Pts',(-43.9829982620799,-76.9144258896296,
21.8947108508307));
#45369=CARTESIAN_POINT('Ctrl Pts',(-43.8785525781174,-78.2292942545683,
22.6506000135548));
#45370=CARTESIAN_POINT('Ctrl Pts',(-43.7841753116354,-79.5742350057765,
22.6486678392791));
#45371=CARTESIAN_POINT('Ctrl Pts',(-43.699672217088,-80.6584337764255,22.1263780555366));
#45372=CARTESIAN_POINT('Ctrl Pts',(-43.6296126732069,-81.2801642158414,
21.3455317785918));
#45373=CARTESIAN_POINT('Ctrl Pts',(-43.5737753994274,-81.5372170176451,
20.6087512726784));
#45374=CARTESIAN_POINT('Ctrl Pts',(-43.518078981982,-81.6250338077328,19.8350853592833));
#45375=CARTESIAN_POINT('Ctrl Pts',(-43.4487183634687,-81.404469536385,18.8724557081866));
#45376=CARTESIAN_POINT('Ctrl Pts',(-43.3658959085869,-80.6687217128354,
17.949784241022));
#45377=CARTESIAN_POINT('Ctrl Pts',(-43.283474596072,-79.610792793437,17.4423031492366));
#45378=CARTESIAN_POINT('Ctrl Pts',(-43.1877734173518,-78.2470216501346,
17.4407977672363));
#45379=CARTESIAN_POINT('Ctrl Pts',(-43.0790453443284,-76.8935395063061,
18.2888255232695));
#45380=CARTESIAN_POINT('Ctrl Pts',(-42.9575637604258,-76.3060155363263,
19.9777434791269));
#45381=CARTESIAN_POINT('Ctrl Pts',(-42.8368801969012,-76.8937775828933,
21.6512107701672));
#45382=CARTESIAN_POINT('Ctrl Pts',(-42.7169622778929,-78.3878970389899,
22.5882669368956));
#45383=CARTESIAN_POINT('Ctrl Pts',(-42.5977722059908,-80.1292261653996,
22.3901838052404));
#45384=CARTESIAN_POINT('Ctrl Pts',(-42.4792718279229,-81.3601746061652,
21.1570532288566));
#45385=CARTESIAN_POINT('Ctrl Pts',(-42.3614218706137,-81.5525719695301,
19.434897660521));
#45386=CARTESIAN_POINT('Ctrl Pts',(-42.2441791418002,-80.6341360625486,
17.9759923568351));
#45387=CARTESIAN_POINT('Ctrl Pts',(-42.1275051232798,-79.0140156775564,
17.4107380824392));
#45388=CARTESIAN_POINT('Ctrl Pts',(-42.0113456022818,-77.4024665017815,
17.9760297721319));
#45389=CARTESIAN_POINT('Ctrl Pts',(-41.8956771393597,-76.4973982517658,
19.41739241847));
#45390=CARTESIAN_POINT('Ctrl Pts',(-41.7804045126007,-76.6899507198097,
21.1009365038956));
#45391=CARTESIAN_POINT('Ctrl Pts',(-41.665545375653,-77.8837303342628,22.2956049805917));
#45392=CARTESIAN_POINT('Ctrl Pts',(-41.5509433179345,-79.5588532573537,
22.4820346193826));
#45393=CARTESIAN_POINT('Ctrl Pts',(-41.4558302779412,-80.7416595080358,
21.73980621753));
#45394=CARTESIAN_POINT('Ctrl Pts',(-41.3795913853863,-81.2587963541492,
20.7938974313728));
#45395=CARTESIAN_POINT('Ctrl Pts',(-41.3417721331875,-81.3480515793144,
20.2756857792622));
#45396=CARTESIAN_POINT('Ctrl Pts',(-41.322588188277,-81.3485521238293,20.0046454119954));
#45397=CARTESIAN_POINT('Ctrl Pts',(-56.5102053539837,-81.351600589951,20.0071836514217));
#45398=CARTESIAN_POINT('Ctrl Pts',(-56.4910244219711,-81.3511001238464,
19.7361858548797));
#45399=CARTESIAN_POINT('Ctrl Pts',(-56.4531917437032,-81.261737846479,19.2178972242685));
#45400=CARTESIAN_POINT('Ctrl Pts',(-56.3770585424072,-80.7451754499662,
18.2734918738261));
#45401=CARTESIAN_POINT('Ctrl Pts',(-56.2823212194466,-79.56681271122,17.5350771162317));
#45402=CARTESIAN_POINT('Ctrl Pts',(-56.168557869964,-77.9044015600755,17.7210078702458));
#45403=CARTESIAN_POINT('Ctrl Pts',(-56.054932665963,-76.7242923839595,18.9032627799536));
#45404=CARTESIAN_POINT('Ctrl Pts',(-55.9412690897771,-76.5353583257392,
20.5629616301326));
#45405=CARTESIAN_POINT('Ctrl Pts',(-55.8275659899422,-77.425346150383,21.9786754829479));
#45406=CARTESIAN_POINT('Ctrl Pts',(-55.7137625672808,-79.0039247999209,
22.5314527230236));
#45407=CARTESIAN_POINT('Ctrl Pts',(-55.5998114833368,-80.5853579566487,
21.9787611516442));
#45408=CARTESIAN_POINT('Ctrl Pts',(-55.4856598482461,-81.4785333921862,
20.5583160012619));
#45409=CARTESIAN_POINT('Ctrl Pts',(-55.3712576510193,-81.2910980626486,
18.8871689581471));
#45410=CARTESIAN_POINT('Ctrl Pts',(-55.2565556248424,-80.0992808803953,
17.6944405340721));
#45411=CARTESIAN_POINT('Ctrl Pts',(-55.141503164892,-78.4192425544493,17.5040643664775));
#45412=CARTESIAN_POINT('Ctrl Pts',(-55.026055868874,-76.9808732902402,18.4064154466049));
#45413=CARTESIAN_POINT('Ctrl Pts',(-54.9294735631935,-76.5128630966309,
19.7455891929516));
#45414=CARTESIAN_POINT('Ctrl Pts',(-54.8519729228635,-76.6978592561223,
20.8220799878041));
#45415=CARTESIAN_POINT('Ctrl Pts',(-54.7937180120044,-77.0938776199365,
21.540591026434));
#45416=CARTESIAN_POINT('Ctrl Pts',(-54.7353290651632,-77.7074901235831,
22.0880670558696));
#45417=CARTESIAN_POINT('Ctrl Pts',(-54.6572920452478,-78.7225626158952,
22.5112243584038));
#45418=CARTESIAN_POINT('Ctrl Pts',(-54.5593711005937,-80.1520967756301,
22.3529289346277));
#45419=CARTESIAN_POINT('Ctrl Pts',(-54.4412482204883,-81.3817174297985,
21.1251765148885));
#45420=CARTESIAN_POINT('Ctrl Pts',(-54.3224612626691,-81.5786773319245,
19.3908351414342));
#45421=CARTESIAN_POINT('Ctrl Pts',(-54.2029675645252,-80.6459478261372,
17.9012773774753));
#45422=CARTESIAN_POINT('Ctrl Pts',(-54.0827425677814,-78.9778893097759,
17.317885726257));
#45423=CARTESIAN_POINT('Ctrl Pts',(-53.9617333429526,-77.2981755739033,
17.9032403007292));
#45424=CARTESIAN_POINT('Ctrl Pts',(-53.8399125595789,-76.3436028630065,
19.4185080130129));
#45425=CARTESIAN_POINT('Ctrl Pts',(-53.7172473194658,-76.5433947171594,
21.2106545999253));
#45426=CARTESIAN_POINT('Ctrl Pts',(-53.5937073203965,-77.8260881060579,
22.4964442551405));
#45427=CARTESIAN_POINT('Ctrl Pts',(-53.4692641471014,-79.6438496446738,
22.7035183202107));
#45428=CARTESIAN_POINT('Ctrl Pts',(-53.3438915061289,-81.2057871862013,
21.7248460212009));
#45429=CARTESIAN_POINT('Ctrl Pts',(-53.2175652348102,-81.8214765038056,
19.9726072217714));
#45430=CARTESIAN_POINT('Ctrl Pts',(-53.0902632570463,-81.2056586657804,
18.2052063703588));
#45431=CARTESIAN_POINT('Ctrl Pts',(-52.9619658262281,-79.6098641790913,
17.1995187197679));
#45432=CARTESIAN_POINT('Ctrl Pts',(-52.8326556330999,-77.7203742313896,
17.4098298281602));
#45433=CARTESIAN_POINT('Ctrl Pts',(-52.7023177766159,-76.3635187904908,
18.7630035707443));
#45434=CARTESIAN_POINT('Ctrl Pts',(-52.570939721051,-76.1446314012751,20.6821481924982));
#45435=CARTESIAN_POINT('Ctrl Pts',(-52.4385113642502,-77.1782614510524,
22.3321665597262));
#45436=CARTESIAN_POINT('Ctrl Pts',(-52.3050249835528,-79.0298407796912,
22.9828907354959));
#45437=CARTESIAN_POINT('Ctrl Pts',(-52.1704753824066,-80.8979297239154,
22.3320439848364));
#45438=CARTESIAN_POINT('Ctrl Pts',(-52.0348597424323,-81.9610122222982,
20.6451414911034));
#45439=CARTESIAN_POINT('Ctrl Pts',(-51.8981780948215,-81.7385564317577,
18.6478788175736));
#45440=CARTESIAN_POINT('Ctrl Pts',(-51.7604321945898,-80.3083549963098,
17.2138695348548));
#45441=CARTESIAN_POINT('Ctrl Pts',(-51.6216279436362,-78.2802930883723,
16.9828845462497));
#45442=CARTESIAN_POINT('Ctrl Pts',(-51.4817699615281,-76.5380718994072,
18.0745070683019));
#45443=CARTESIAN_POINT('Ctrl Pts',(-51.3408736679231,-75.8501788412933,
20.0297405359875));
#45444=CARTESIAN_POINT('Ctrl Pts',(-51.1989382729077,-76.5392195094218,
21.9991175294759));
#45445=CARTESIAN_POINT('Ctrl Pts',(-51.0559946652494,-78.3171890144164,
23.1196650869329));
#45446=CARTESIAN_POINT('Ctrl Pts',(-50.9120515053575,-80.4205653742962,
22.8851695343114));
#45447=CARTESIAN_POINT('Ctrl Pts',(-50.7671291242161,-81.9289478457697,
21.380149508053));
#45448=CARTESIAN_POINT('Ctrl Pts',(-50.6212487099078,-82.1713186731815,
19.248852229337));
#45449=CARTESIAN_POINT('Ctrl Pts',(-50.474433980975,-81.0247130386606,17.4198125584412));
#45450=CARTESIAN_POINT('Ctrl Pts',(-50.3267111772793,-78.9748712348568,
16.7000982510701));
#45451=CARTESIAN_POINT('Ctrl Pts',(-50.1781079176229,-76.9120299405903,
17.420093293127));
#45452=CARTESIAN_POINT('Ctrl Pts',(-50.0286560537834,-75.7398510408867,
19.2788548996711));
#45453=CARTESIAN_POINT('Ctrl Pts',(-49.8783844328933,-75.9874937562904,
21.476647216806));
#45454=CARTESIAN_POINT('Ctrl Pts',(-49.7273345651342,-77.5512046364284,
23.0443219045335));
#45455=CARTESIAN_POINT('Ctrl Pts',(-49.5586585240247,-80.0279089996088,
23.3334401353208));
#45456=CARTESIAN_POINT('Ctrl Pts',(-49.4060082642688,-81.8538210133292,
21.8837856461858));
#45457=CARTESIAN_POINT('Ctrl Pts',(-49.2782581021314,-82.2484807046217,
20.0963040292974));
#45458=CARTESIAN_POINT('Ctrl Pts',(-49.1928885669734,-82.0489182365846,
18.914665854516));
#45459=CARTESIAN_POINT('Ctrl Pts',(-49.0902384690458,-81.3507219395805,
17.6452269478581));
#45460=CARTESIAN_POINT('Ctrl Pts',(-48.9615765066383,-79.7525096231734,
16.6379188946829));
#45461=CARTESIAN_POINT('Ctrl Pts',(-48.8066280268286,-77.4866354369491,
16.8915282252642));
#45462=CARTESIAN_POINT('Ctrl Pts',(-48.6511833135857,-75.870236297486,18.5070672541726));
#45463=CARTESIAN_POINT('Ctrl Pts',(-48.4952829185379,-75.6121761854611,
20.7849669355286));
#45464=CARTESIAN_POINT('Ctrl Pts',(-48.3389764832945,-76.8343636892977,
22.731649389924));
#45465=CARTESIAN_POINT('Ctrl Pts',(-48.1823111553132,-79.0084616600531,
23.4933056118749));
#45466=CARTESIAN_POINT('Ctrl Pts',(-48.0253367390954,-81.1874456640624,
22.7316029756924));
#45467=CARTESIAN_POINT('Ctrl Pts',(-47.8681030052212,-82.4179904745334,
20.7742238673546));
#45468=CARTESIAN_POINT('Ctrl Pts',(-47.7106605343791,-82.1591871711449,
18.4735616689089));
#45469=CARTESIAN_POINT('Ctrl Pts',(-47.5530598605685,-80.5206179988346,
16.8346671108224));
#45470=CARTESIAN_POINT('Ctrl Pts',(-47.3953525426489,-78.2160956239723,
16.5747442943651));
#45471=CARTESIAN_POINT('Ctrl Pts',(-47.2375889524593,-76.2515474551307,
17.8091507733092));
#45472=CARTESIAN_POINT('Ctrl Pts',(-47.0798232077956,-75.48537779457,19.9985379877705));
#45473=CARTESIAN_POINT('Ctrl Pts',(-46.9221018381816,-76.250966995779,22.1885862850942));
#45474=CARTESIAN_POINT('Ctrl Pts',(-46.7907582490246,-77.887069828226,23.2141549060391));
#45475=CARTESIAN_POINT('Ctrl Pts',(-46.6857437519368,-79.3633599628629,
23.2931678430071));
#45476=CARTESIAN_POINT('Ctrl Pts',(-46.5807886964194,-80.7886728129746,
22.8877056847724));
#45477=CARTESIAN_POINT('Ctrl Pts',(-46.467199813299,-81.9623024203698,21.7095989845971));
#45478=CARTESIAN_POINT('Ctrl Pts',(-46.3101244066264,-82.4667648192415,
19.5204885422792));
#45479=CARTESIAN_POINT('Ctrl Pts',(-46.1990680734046,-81.7418829913271,
17.9904302358176));
#45480=CARTESIAN_POINT('Ctrl Pts',(-46.1164515816408,-80.8095926681598,
17.3151909175046));
#45481=CARTESIAN_POINT('Ctrl Pts',(-46.0642853611533,-80.1910909998415,
16.9374483432803));
#45482=CARTESIAN_POINT('Ctrl Pts',(-45.9665775630929,-78.8344213924405,
16.5853757174044));
#45483=CARTESIAN_POINT('Ctrl Pts',(-45.8236196285692,-76.8476963089672,
17.2805323474208));
#45484=CARTESIAN_POINT('Ctrl Pts',(-45.668075484254,-75.6358728708552,19.2140995275267));
#45485=CARTESIAN_POINT('Ctrl Pts',(-45.4958299283901,-75.9121578661318,
21.7421177773414));
#45486=CARTESIAN_POINT('Ctrl Pts',(-45.3242577516971,-77.9692102287361,
23.38035508761));
#45487=CARTESIAN_POINT('Ctrl Pts',(-45.1876221856116,-79.9670552350402,
23.139500775403));
#45488=CARTESIAN_POINT('Ctrl Pts',(-45.0513558128287,-81.5832325086694,
22.1319648181091));
#45489=CARTESIAN_POINT('Ctrl Pts',(-44.8986075069025,-82.5974332632258,
20.0161637774792));
#45490=CARTESIAN_POINT('Ctrl Pts',(-44.7186795070239,-81.3925086591267,
17.5302291648947));
#45491=CARTESIAN_POINT('Ctrl Pts',(-44.5621230479846,-79.2651609763857,
16.712655372227));
#45492=CARTESIAN_POINT('Ctrl Pts',(-44.4285417889314,-77.3774483800612,
17.139881442109));
#45493=CARTESIAN_POINT('Ctrl Pts',(-44.2956173863613,-76.0640042276617,
18.5597990145458));
#45494=CARTESIAN_POINT('Ctrl Pts',(-44.1633484646108,-75.7783293923941,
20.4582768445098));
#45495=CARTESIAN_POINT('Ctrl Pts',(-44.031779218605,-76.6099851009247,22.1814794461785));
#45496=CARTESIAN_POINT('Ctrl Pts',(-43.91182076343,-78.1200466389143,23.0500041168154));
#45497=CARTESIAN_POINT('Ctrl Pts',(-43.8032972503512,-79.6666485186877,
23.0479392254152));
#45498=CARTESIAN_POINT('Ctrl Pts',(-43.7060427882043,-80.9145301144203,
22.4469274515336));
#45499=CARTESIAN_POINT('Ctrl Pts',(-43.6253519025163,-81.6306856242157,
21.5476182586661));
#45500=CARTESIAN_POINT('Ctrl Pts',(-43.5610123031743,-81.9268920837325,
20.6986435448477));
#45501=CARTESIAN_POINT('Ctrl Pts',(-43.4968178170664,-82.0281189549035,
19.806937944391));
#45502=CARTESIAN_POINT('Ctrl Pts',(-43.4168479041046,-81.7738600390164,
18.6970519690361));
#45503=CARTESIAN_POINT('Ctrl Pts',(-43.3213263793924,-80.9253416906861,
17.6329077834861));
#45504=CARTESIAN_POINT('Ctrl Pts',(-43.2262532956317,-79.7050475580838,
17.0475327158774));
#45505=CARTESIAN_POINT('Ctrl Pts',(-43.1158616470016,-78.1319653479767,
17.0458078617628));
#45506=CARTESIAN_POINT('Ctrl Pts',(-42.9904623873872,-76.5711141945366,
18.0239064285819));
#45507=CARTESIAN_POINT('Ctrl Pts',(-42.8504284292441,-75.8942100281233,
19.9706479680719));
#45508=CARTESIAN_POINT('Ctrl Pts',(-42.7114451655225,-76.5714158474922,
21.8975344967549));
#45509=CARTESIAN_POINT('Ctrl Pts',(-42.5735200918022,-78.2899803626415,
22.9747252284951));
#45510=CARTESIAN_POINT('Ctrl Pts',(-42.4366584097288,-80.2891630255458,
22.7466550039197));
#45511=CARTESIAN_POINT('Ctrl Pts',(-42.300862738502,-81.6990410530149,21.3332139952526));
#45512=CARTESIAN_POINT('Ctrl Pts',(-42.1661332961441,-81.9181163628249,
19.3646257221592));
#45513=CARTESIAN_POINT('Ctrl Pts',(-42.0324677389737,-80.8704178528976,
17.7021871370045));
#45514=CARTESIAN_POINT('Ctrl Pts',(-41.8998614427592,-79.0291889851441,
17.060906941546));
#45515=CARTESIAN_POINT('Ctrl Pts',(-41.768306817613,-77.204873422229,17.7021299380875));
#45516=CARTESIAN_POINT('Ctrl Pts',(-41.6377947505436,-76.1852713423579,
19.3284903687226));
#45517=CARTESIAN_POINT('Ctrl Pts',(-41.5083116255931,-76.4029798468466,
21.2192502585522));
#45518=CARTESIAN_POINT('Ctrl Pts',(-41.3798598292886,-77.7388493644985,
22.5535329081885));
#45519=CARTESIAN_POINT('Ctrl Pts',(-41.252378015881,-79.6025795576068,22.7597660265109));
#45520=CARTESIAN_POINT('Ctrl Pts',(-41.1470144444954,-80.9111847600037,
21.93603750269));
#45521=CARTESIAN_POINT('Ctrl Pts',(-41.0631067409177,-81.4804422184361,
20.8951581990914));
#45522=CARTESIAN_POINT('Ctrl Pts',(-41.0214391827265,-81.5786120505805,
20.3242243526537));
#45523=CARTESIAN_POINT('Ctrl Pts',(-41.0004636061353,-81.5791593420714,
20.0278709170366));
#45524=CARTESIAN_POINT('Ctrl Pts',(-56.1931710509147,-81.5904762192943,
20.0291818533745));
#45525=CARTESIAN_POINT('Ctrl Pts',(-56.1721965566912,-81.5899289558238,
19.7328437132649));
#45526=CARTESIAN_POINT('Ctrl Pts',(-56.1304803139095,-81.4914160150344,
19.1612770147036));
#45527=CARTESIAN_POINT('Ctrl Pts',(-56.047109678892,-80.9249724047485,18.1271447389076));
#45528=CARTESIAN_POINT('Ctrl Pts',(-55.9436715369273,-79.6379237377103,
17.3216367798175));
#45529=CARTESIAN_POINT('Ctrl Pts',(-55.8203317637762,-77.8351613950806,
17.5256562815028));
#45530=CARTESIAN_POINT('Ctrl Pts',(-55.69790582868,-76.5650422099848,18.8008040261662));
#45531=CARTESIAN_POINT('Ctrl Pts',(-55.5762992644413,-76.3649861666019,
20.5773747368897));
#45532=CARTESIAN_POINT('Ctrl Pts',(-55.4555213165667,-77.312671536182,22.0805289509775));
#45533=CARTESIAN_POINT('Ctrl Pts',(-55.3355023408405,-78.9788215337353,
22.661615143053));
#45534=CARTESIAN_POINT('Ctrl Pts',(-55.2162218985695,-80.6341462766125,
22.0806902291229));
#45535=CARTESIAN_POINT('Ctrl Pts',(-55.0976344395572,-81.5604707585099,
20.6032956261243));
#45536=CARTESIAN_POINT('Ctrl Pts',(-54.9797037858124,-81.3649349503641,
18.8802080061892));
#45537=CARTESIAN_POINT('Ctrl Pts',(-54.8623863490237,-80.1439213865375,
17.6614773952729));
#45538=CARTESIAN_POINT('Ctrl Pts',(-54.7456423816505,-78.438301885998,17.4704950427283));
#45539=CARTESIAN_POINT('Ctrl Pts',(-54.6294225574966,-76.9911289094193,
18.381155317716));
#45540=CARTESIAN_POINT('Ctrl Pts',(-54.5329814401706,-76.5254042740319,
19.719510916299));
#45541=CARTESIAN_POINT('Ctrl Pts',(-54.4560325840395,-76.709489835983,20.788354755425));
#45542=CARTESIAN_POINT('Ctrl Pts',(-54.3984251024622,-77.1014268283988,
21.4989031483612));
#45543=CARTESIAN_POINT('Ctrl Pts',(-54.3409144108848,-77.7060790817609,
22.0380321813387));
#45544=CARTESIAN_POINT('Ctrl Pts',(-54.2643529957864,-78.7023284793725,
22.4529267891116));
#45545=CARTESIAN_POINT('Ctrl Pts',(-54.1688795115049,-80.0965435535358,
22.2967139321817));
#45546=CARTESIAN_POINT('Ctrl Pts',(-54.0545941116151,-81.2849959119691,
21.1068835663603));
#45547=CARTESIAN_POINT('Ctrl Pts',(-53.9405474572273,-81.4719923932769,
19.441012695379));
#45548=CARTESIAN_POINT('Ctrl Pts',(-53.8266972060701,-80.5811209890118,
18.0223892278746));
#45549=CARTESIAN_POINT('Ctrl Pts',(-53.7129653055039,-79.0022844568973,
17.472401568245));
#45550=CARTESIAN_POINT('Ctrl Pts',(-53.599334468734,-77.4251558030463,18.0241320621135));
#45551=CARTESIAN_POINT('Ctrl Pts',(-53.4857367540597,-76.5364154437238,
19.4385659324685));
#45552=CARTESIAN_POINT('Ctrl Pts',(-53.3721220169306,-76.7233926686843,
21.0987319736096));
#45553=CARTESIAN_POINT('Ctrl Pts',(-53.2584384574455,-77.9053472090669,
22.2809672747817));
#45554=CARTESIAN_POINT('Ctrl Pts',(-53.1446349951865,-79.568314662251,22.4686541503725));
#45555=CARTESIAN_POINT('Ctrl Pts',(-53.030660482889,-80.9877176287472,21.577332089441));
#45556=CARTESIAN_POINT('Ctrl Pts',(-52.9164642736675,-81.5429354152238,
19.9924518303138));
#45557=CARTESIAN_POINT('Ctrl Pts',(-52.8019958227748,-80.9876773944488,
18.4033565400404));
#45558=CARTESIAN_POINT('Ctrl Pts',(-52.6872052811913,-79.5588434690807,
17.5045277438755));
#45559=CARTESIAN_POINT('Ctrl Pts',(-52.5720437782595,-77.8759033624557,
17.6931479297474));
#45560=CARTESIAN_POINT('Ctrl Pts',(-52.456463479153,-76.6732981208235,18.8941780160138));
#45561=CARTESIAN_POINT('Ctrl Pts',(-52.3404174742245,-76.4810117294207,
20.5897747255326));
#45562=CARTESIAN_POINT('Ctrl Pts',(-52.2238599700478,-77.3917589649615,
22.0417537639404));
#45563=CARTESIAN_POINT('Ctrl Pts',(-52.1067461880084,-79.0167757404078,
22.6119079176574));
#45564=CARTESIAN_POINT('Ctrl Pts',(-51.9890325238844,-80.6510816764256,
22.0416788272352));
#45565=CARTESIAN_POINT('Ctrl Pts',(-51.8706765682083,-81.5784074709173,
20.5689210739554));
#45566=CARTESIAN_POINT('Ctrl Pts',(-51.7516381842611,-81.3840761178566,
18.8293385290052));
#45567=CARTESIAN_POINT('Ctrl Pts',(-51.6318777612795,-80.1401644139924,
17.5827772497869));
#45568=CARTESIAN_POINT('Ctrl Pts',(-51.5113598466867,-78.3790893485887,
17.3825631025712));
#45569=CARTESIAN_POINT('Ctrl Pts',(-51.3900453226883,-76.8679002321331,
18.3297321532828));
#45570=CARTESIAN_POINT('Ctrl Pts',(-51.2679089636746,-76.2716995874448,
20.0248007634938));
#45571=CARTESIAN_POINT('Ctrl Pts',(-51.1448999383953,-76.8689071318202,
21.731599205865));
#45572=CARTESIAN_POINT('Ctrl Pts',(-51.021010641651,-78.4098824882715,22.7028590477005));
#45573=CARTESIAN_POINT('Ctrl Pts',(-50.8962035466111,-80.2336798734102,
22.4997020368517));
#45574=CARTESIAN_POINT('Ctrl Pts',(-50.7704540538976,-81.5427020047577,
21.1939832796085));
#45575=CARTESIAN_POINT('Ctrl Pts',(-50.6437387988144,-81.753601597011,19.3427496141414));
#45576=CARTESIAN_POINT('Ctrl Pts',(-50.5160369129462,-80.7566939083138,
17.7516096622113));
#45577=CARTESIAN_POINT('Ctrl Pts',(-50.3873296992986,-78.9709799251651,
17.1240176730073));
#45578=CARTESIAN_POINT('Ctrl Pts',(-50.2576005805652,-77.1700135782155,
17.75191180977));
#45579=CARTESIAN_POINT('Ctrl Pts',(-50.1268359834938,-76.1438312789394,
19.3777143443819));
#45580=CARTESIAN_POINT('Ctrl Pts',(-49.9950235011709,-76.3601822381745,
21.3055450852728));
#45581=CARTESIAN_POINT('Ctrl Pts',(-49.8621562390858,-77.7348938688194,
22.6849411190031));
#45582=CARTESIAN_POINT('Ctrl Pts',(-49.7133415381469,-79.9195947555483,
22.9413584111036));
#45583=CARTESIAN_POINT('Ctrl Pts',(-49.5781602668827,-81.5376672860394,
21.6590948623266));
#45584=CARTESIAN_POINT('Ctrl Pts',(-49.4646197181616,-81.8890632572599,
20.0705481237758));
#45585=CARTESIAN_POINT('Ctrl Pts',(-49.3885799052481,-81.7114130509256,
19.0181107772552));
#45586=CARTESIAN_POINT('Ctrl Pts',(-49.2969766628829,-81.0886388482757,
17.8852892572052));
#45587=CARTESIAN_POINT('Ctrl Pts',(-49.181806776448,-79.6588985177388,16.9828625133814));
#45588=CARTESIAN_POINT('Ctrl Pts',(-49.0425442242264,-77.6225755834458,
17.2092920570815));
#45589=CARTESIAN_POINT('Ctrl Pts',(-48.9022309275819,-76.1626933241173,
18.6662194328442));
#45590=CARTESIAN_POINT('Ctrl Pts',(-48.7608776813598,-75.9271678115608,
20.7310072076683));
#45591=CARTESIAN_POINT('Ctrl Pts',(-48.6184974980409,-77.038831411295,22.5047935543629));
#45592=CARTESIAN_POINT('Ctrl Pts',(-48.4751059278121,-79.0277630066599,
23.2034124271523));
#45593=CARTESIAN_POINT('Ctrl Pts',(-48.3307209130028,-81.0321747592271,
22.5046334535624));
#45594=CARTESIAN_POINT('Ctrl Pts',(-48.1853628100416,-82.1711101595149,
20.6964577220007));
#45595=CARTESIAN_POINT('Ctrl Pts',(-48.0390540416698,-81.9325628945093,
18.5587419776551));
#45596=CARTESIAN_POINT('Ctrl Pts',(-47.8918194155008,-80.4035068057025,
17.0266017125607));
#45597=CARTESIAN_POINT('Ctrl Pts',(-47.7436853224969,-78.2396309977359,
16.7805121138364));
#45598=CARTESIAN_POINT('Ctrl Pts',(-47.5946813664555,-76.3835179295052,
17.9443525134594));
#45599=CARTESIAN_POINT('Ctrl Pts',(-47.4448367983989,-75.6540675159799,
20.02254637128));
#45600=CARTESIAN_POINT('Ctrl Pts',(-47.2941883295031,-76.3830994404273,
22.114567621428));
#45601=CARTESIAN_POINT('Ctrl Pts',(-47.1679999676535,-77.9535609675346,
23.1010714787732));
#45602=CARTESIAN_POINT('Ctrl Pts',(-47.0666921451397,-79.3776145525847,
23.1776099822803));
#45603=CARTESIAN_POINT('Ctrl Pts',(-46.9651456325947,-80.7564776023867,
22.7858153407833));
#45604=CARTESIAN_POINT('Ctrl Pts',(-46.8547566881906,-81.8978095452959,
21.6420721310674));
#45605=CARTESIAN_POINT('Ctrl Pts',(-46.7013715271651,-82.3915913662202,
19.5050054644041));
#45606=CARTESIAN_POINT('Ctrl Pts',(-46.5922746342819,-81.6820066722275,
18.0013720242213));
#45607=CARTESIAN_POINT('Ctrl Pts',(-46.5107702934997,-80.762347045538,17.3351375612649));
#45608=CARTESIAN_POINT('Ctrl Pts',(-46.4592725150514,-80.1518069976578,
16.962269556289));
#45609=CARTESIAN_POINT('Ctrl Pts',(-46.362556488097,-78.8093578228561,16.6130383905039));
#45610=CARTESIAN_POINT('Ctrl Pts',(-46.220252885875,-76.8319457334074,17.3026718943654));
#45611=CARTESIAN_POINT('Ctrl Pts',(-46.0645726816584,-75.6173234870341,
19.2366771428804));
#45612=CARTESIAN_POINT('Ctrl Pts',(-45.8910714666791,-75.8925338508242,
21.7821315892937));
#45613=CARTESIAN_POINT('Ctrl Pts',(-45.7170955988033,-77.9753043773735,
23.4465775524674));
#45614=CARTESIAN_POINT('Ctrl Pts',(-45.5775759501255,-80.0153755859992,
23.2028167937863));
#45615=CARTESIAN_POINT('Ctrl Pts',(-45.4379062168885,-81.6717237264668,
22.1705201271916));
#45616=CARTESIAN_POINT('Ctrl Pts',(-45.2805526561883,-82.7200865632941,
19.9931079900749));
#45617=CARTESIAN_POINT('Ctrl Pts',(-45.0937704500736,-81.4738598243379,
17.4107654017481));
#45618=CARTESIAN_POINT('Ctrl Pts',(-44.9301776981165,-79.2519774158652,
16.5546323280892));
#45619=CARTESIAN_POINT('Ctrl Pts',(-44.7899176784637,-77.2699004358815,
17.0018364132725));
#45620=CARTESIAN_POINT('Ctrl Pts',(-44.6496109849249,-75.8827842307996,
18.4989471414362));
#45621=CARTESIAN_POINT('Ctrl Pts',(-44.5093442071425,-75.5784269695796,
20.5118097310074));
#45622=CARTESIAN_POINT('Ctrl Pts',(-44.3691027049655,-76.4632134679003,
22.3486394697955));
#45623=CARTESIAN_POINT('Ctrl Pts',(-44.2406353839749,-78.0793884615202,
23.2797044070866));
#45624=CARTESIAN_POINT('Ctrl Pts',(-44.1239394431124,-79.7421639402498,
23.2781543264229));
#45625=CARTESIAN_POINT('Ctrl Pts',(-44.0189993614293,-81.0886776635895,
22.6302737684353));
#45626=CARTESIAN_POINT('Ctrl Pts',(-43.9316263801741,-81.8643428824872,
21.6570022286492));
#45627=CARTESIAN_POINT('Ctrl Pts',(-43.8617948533705,-82.1859028857951,
20.7356337027876));
#45628=CARTESIAN_POINT('Ctrl Pts',(-43.7920004881958,-82.2960384222753,
19.7662775164889));
#45629=CARTESIAN_POINT('Ctrl Pts',(-43.7048391513216,-82.0193817005433,
18.5565903493298));
#45630=CARTESIAN_POINT('Ctrl Pts',(-43.6003869534277,-81.0920630654462,
17.3927421594966));
#45631=CARTESIAN_POINT('Ctrl Pts',(-43.4960916257064,-79.7537507355311,
16.7501788420722));
#45632=CARTESIAN_POINT('Ctrl Pts',(-43.3746208877838,-78.0229433571945,
16.7476551770101));
#45633=CARTESIAN_POINT('Ctrl Pts',(-43.2360946688018,-76.2982193406305,
17.8266391512518));
#45634=CARTESIAN_POINT('Ctrl Pts',(-43.0807103498632,-75.5455686337531,
19.9858138830528));
#45635=CARTESIAN_POINT('Ctrl Pts',(-42.9258436987913,-76.2985455065884,
22.1331261217648));
#45636=CARTESIAN_POINT('Ctrl Pts',(-42.77153307093,-78.2201494104768,23.3393944253305));
#45637=CARTESIAN_POINT('Ctrl Pts',(-42.6178242859543,-80.4652865043261,
23.0847085443991));
#45638=CARTESIAN_POINT('Ctrl Pts',(-42.4647580213375,-82.0552277538098,
21.4926381936908));
#45639=CARTESIAN_POINT('Ctrl Pts',(-42.3123743467156,-82.3042292356101,
19.2664619793303));
#45640=CARTESIAN_POINT('Ctrl Pts',(-42.1607129706379,-81.1165722086679,
17.3797443302913));
#45641=CARTESIAN_POINT('Ctrl Pts',(-42.0098077521494,-79.0218319254807,
16.6489801585146));
#45642=CARTESIAN_POINT('Ctrl Pts',(-41.8597011624017,-76.9400588245036,
17.3796589230168));
#45643=CARTESIAN_POINT('Ctrl Pts',(-41.710410410155,-75.7731819376884,19.2391358645968));
#45644=CARTESIAN_POINT('Ctrl Pts',(-41.5620024200472,-76.021931806847,21.4065209298965));
#45645=CARTESIAN_POINT('Ctrl Pts',(-41.41446762267,-77.5555540696917,22.938792418932));
#45646=CARTESIAN_POINT('Ctrl Pts',(-41.267888073828,-79.69889898891,23.1771584642698));
#45647=CARTESIAN_POINT('Ctrl Pts',(-41.1464403049599,-81.2063623988802,
22.2273394788785));
#45648=CARTESIAN_POINT('Ctrl Pts',(-41.049904311213,-81.8619881545566,21.0300427262042));
#45649=CARTESIAN_POINT('Ctrl Pts',(-41.0016934823989,-81.975435692595,20.3694323176616));
#45650=CARTESIAN_POINT('Ctrl Pts',(-40.977684131746,-81.9760621408481,20.030216204962));
#45651=CARTESIAN_POINT('Ctrl Pts',(-56.1840163481737,-81.9875883200479,
20.0290964452435));
#45652=CARTESIAN_POINT('Ctrl Pts',(-56.1600105776776,-81.9869619649552,
19.6899309185389));
#45653=CARTESIAN_POINT('Ctrl Pts',(-56.1117529637962,-81.8731652833032,
19.0287333656979));
#45654=CARTESIAN_POINT('Ctrl Pts',(-56.0157840520367,-81.2205270484806,
17.8385771112663));
#45655=CARTESIAN_POINT('Ctrl Pts',(-55.896346951956,-79.7356206089475,16.9078031975861));
#45656=CARTESIAN_POINT('Ctrl Pts',(-55.7540857207524,-77.6558823397947,
17.1438436556406));
#45657=CARTESIAN_POINT('Ctrl Pts',(-55.6128283938031,-76.1907775976361,
18.6144681707804));
#45658=CARTESIAN_POINT('Ctrl Pts',(-55.4726208861106,-75.9604020090565,
20.6628992338605));
#45659=CARTESIAN_POINT('Ctrl Pts',(-55.3334578707361,-77.0523722890483,
22.3940848262856));
#45660=CARTESIAN_POINT('Ctrl Pts',(-55.1953542744678,-78.9694706157036,
23.0621619556173));
#45661=CARTESIAN_POINT('Ctrl Pts',(-55.0583124323056,-80.8706958719993,
22.3942275308775));
#45662=CARTESIAN_POINT('Ctrl Pts',(-54.9223368518524,-81.9320218793108,
20.7000997936462));
#45663=CARTESIAN_POINT('Ctrl Pts',(-54.7874272612403,-81.7075151506292,
18.7294034487537));
#45664=CARTESIAN_POINT('Ctrl Pts',(-54.6535823409156,-80.3140723860071,
17.3399419744697));
#45665=CARTESIAN_POINT('Ctrl Pts',(-54.5207967868566,-78.374400120103,17.1238400380949));
#45666=CARTESIAN_POINT('Ctrl Pts',(-54.3890655740886,-76.7350629052144,
18.1568592070291));
#45667=CARTESIAN_POINT('Ctrl Pts',(-54.2801569414996,-76.2103002516481,
19.668090987021));
#45668=CARTESIAN_POINT('Ctrl Pts',(-54.1935510059906,-76.4176946207056,
20.8708526855492));
#45669=CARTESIAN_POINT('Ctrl Pts',(-54.128852397298,-76.857964212694,21.6686798646502));
#45670=CARTESIAN_POINT('Ctrl Pts',(-54.0644082411501,-77.5355178162316,
22.2725716773656));
#45671=CARTESIAN_POINT('Ctrl Pts',(-53.9788200417259,-78.6492334202541,
22.7361008606065));
#45672=CARTESIAN_POINT('Ctrl Pts',(-53.8724521289787,-80.2018795945108,
22.5608064996248));
#45673=CARTESIAN_POINT('Ctrl Pts',(-53.7457963218449,-81.5173535677004,
21.2413375034754));
#45674=CARTESIAN_POINT('Ctrl Pts',(-53.6201029336044,-81.721643630464,19.4056787875082));
#45675=CARTESIAN_POINT('Ctrl Pts',(-53.4953423172526,-80.7441720245738,
17.8527194339666));
#45676=CARTESIAN_POINT('Ctrl Pts',(-53.3715075050393,-79.024792546053,17.2558018189766));
#45677=CARTESIAN_POINT('Ctrl Pts',(-53.2485467601093,-77.3194469011662,
17.8545268954824));
#45678=CARTESIAN_POINT('Ctrl Pts',(-53.1264418459081,-76.3662466418217,
19.3754622160036));
#45679=CARTESIAN_POINT('Ctrl Pts',(-53.005159492876,-76.5678911164086,21.1467949273089));
#45680=CARTESIAN_POINT('Ctrl Pts',(-52.8846665013463,-77.8217327869644,
22.3978467499115));
#45681=CARTESIAN_POINT('Ctrl Pts',(-52.7649271902849,-79.5710431464096,
22.5930405834681));
#45682=CARTESIAN_POINT('Ctrl Pts',(-52.6459043559135,-81.0515632714903,
21.6606738718825));
#45683=CARTESIAN_POINT('Ctrl Pts',(-52.527559012935,-81.6245808941478,20.0180744750991));
#45684=CARTESIAN_POINT('Ctrl Pts',(-52.4098503630411,-81.0516487109053,
18.3853810869962));
#45685=CARTESIAN_POINT('Ctrl Pts',(-52.2927360961711,-79.59321937671,17.4706707303658));
#45686=CARTESIAN_POINT('Ctrl Pts',(-52.1761727220418,-77.8907123681399,
17.6638192609241));
#45687=CARTESIAN_POINT('Ctrl Pts',(-52.0601156179322,-76.6852554675414,
18.870974293838));
#45688=CARTESIAN_POINT('Ctrl Pts',(-51.9445189762202,-76.4960826665638,
20.5596055972846));
#45689=CARTESIAN_POINT('Ctrl Pts',(-51.8293359020739,-77.3976800945512,
21.99268490099));
#45690=CARTESIAN_POINT('Ctrl Pts',(-51.7145184824162,-78.9909626260138,
22.5493032765671));
#45691=CARTESIAN_POINT('Ctrl Pts',(-51.6000175219678,-80.5793083717327,
21.9927446344126));
#45692=CARTESIAN_POINT('Ctrl Pts',(-51.4857834151221,-81.4721331834413,
20.5706570604428));
#45693=CARTESIAN_POINT('Ctrl Pts',(-51.3717654497242,-81.2839320663009,
18.9053328706095));
#45694=CARTESIAN_POINT('Ctrl Pts',(-51.2579142567362,-80.1003468389221,
17.7222119598947));
#45695=CARTESIAN_POINT('Ctrl Pts',(-51.1441760738262,-78.4387785300752,
17.5353834584123));
#45696=CARTESIAN_POINT('Ctrl Pts',(-51.0305059559029,-77.0243269868296,
18.4242496721567));
#45697=CARTESIAN_POINT('Ctrl Pts',(-50.9168383295718,-76.4715635155443,
20.0017362886162));
#45698=CARTESIAN_POINT('Ctrl Pts',(-50.8031528501867,-77.0251058898071,
21.5782322028432));
#45699=CARTESIAN_POINT('Ctrl Pts',(-50.6893600620005,-78.4409437964808,
22.4685167016839));
#45700=CARTESIAN_POINT('Ctrl Pts',(-50.5754265208159,-80.1051012370473,
22.281444116521));
#45701=CARTESIAN_POINT('Ctrl Pts',(-50.4612995336001,-81.2916130994061,
21.0956690984439));
#45702=CARTESIAN_POINT('Ctrl Pts',(-50.3469292478256,-81.4804026348622,
19.4251616901667));
#45703=CARTESIAN_POINT('Ctrl Pts',(-50.2322658318771,-80.5843542802,17.9976877444011));
#45704=CARTESIAN_POINT('Ctrl Pts',(-50.1172596710639,-78.9887878135073,
17.4383486295407));
#45705=CARTESIAN_POINT('Ctrl Pts',(-50.0018627971402,-77.3876668209355,
17.9978807978644));
#45706=CARTESIAN_POINT('Ctrl Pts',(-49.8860256103752,-76.4798823834744,
19.4383054994183));
#45707=CARTESIAN_POINT('Ctrl Pts',(-49.7697055460028,-76.6717902993605,
21.1389672456695));
#45708=CARTESIAN_POINT('Ctrl Pts',(-49.6528483461859,-77.8811686925252,
22.3512019911516));
#45709=CARTESIAN_POINT('Ctrl Pts',(-49.5223825436566,-79.7962746252137,
22.5748992760119));
#45710=CARTESIAN_POINT('Ctrl Pts',(-49.4042570362098,-81.2094493464976,
21.4535078840428));
#45711=CARTESIAN_POINT('Ctrl Pts',(-49.3052520376841,-81.5155121502254,
20.0685103690615));
#45712=CARTESIAN_POINT('Ctrl Pts',(-49.2390213385448,-81.3607622132748,
19.1519212626098));
#45713=CARTESIAN_POINT('Ctrl Pts',(-49.1593082369371,-80.8187609382315,
18.1662414366685));
#45714=CARTESIAN_POINT('Ctrl Pts',(-49.0591919240773,-79.5759523510137,
17.3821693816316));
#45715=CARTESIAN_POINT('Ctrl Pts',(-48.9382874011232,-77.8082989807897,
17.5790252757248));
#45716=CARTESIAN_POINT('Ctrl Pts',(-48.8165729896642,-76.5422165483546,
18.8427933888379));
#45717=CARTESIAN_POINT('Ctrl Pts',(-48.6940204727097,-76.3381158557561,
20.6327850920547));
#45718=CARTESIAN_POINT('Ctrl Pts',(-48.5705971077618,-77.3016688744965,
22.1702805692189));
#45719=CARTESIAN_POINT('Ctrl Pts',(-48.4462749687256,-79.0259411160725,
22.7760661916481));
#45720=CARTESIAN_POINT('Ctrl Pts',(-48.3210268594155,-80.7646781227256,
22.1701438364573));
#45721=CARTESIAN_POINT('Ctrl Pts',(-48.194828354645,-81.7537397700009,20.600520392927));
#45722=CARTESIAN_POINT('Ctrl Pts',(-48.067657124948,-81.5468220181871,18.7423903191848));
#45723=CARTESIAN_POINT('Ctrl Pts',(-47.939493283709,-80.2161779802247,17.408315588859));
#45724=CARTESIAN_POINT('Ctrl Pts',(-47.8103191852242,-78.3292737794169,
17.1930918886314));
#45725=CARTESIAN_POINT('Ctrl Pts',(-47.6801196014556,-76.7069354904978,
18.2094845308307));
#45726=CARTESIAN_POINT('Ctrl Pts',(-47.5488814434326,-76.0672383673362,
20.0294810068135));
#45727=CARTESIAN_POINT('Ctrl Pts',(-47.416594505357,-76.7065669191,21.8669523450674));
#45728=CARTESIAN_POINT('Ctrl Pts',(-47.3054739921019,-78.0892405398055,
22.7364966500394));
#45729=CARTESIAN_POINT('Ctrl Pts',(-47.2160471510534,-79.3463826256051,
22.8042334163218));
#45730=CARTESIAN_POINT('Ctrl Pts',(-47.1262652329036,-80.5655791894923,
22.4580413955535));
#45731=CARTESIAN_POINT('Ctrl Pts',(-47.028424926471,-81.5778068418593,21.4447201314267));
#45732=CARTESIAN_POINT('Ctrl Pts',(-46.8920633743752,-82.0174655355277,
19.5449713709624));
#45733=CARTESIAN_POINT('Ctrl Pts',(-46.7947208039299,-81.3856409780859,
18.2026916859546));
#45734=CARTESIAN_POINT('Ctrl Pts',(-46.7217816589043,-80.5625621836747,
17.6063431295216));
#45735=CARTESIAN_POINT('Ctrl Pts',(-46.6756703161032,-80.0158736768733,
17.2724754919093));
#45736=CARTESIAN_POINT('Ctrl Pts',(-46.5889231063328,-78.8118838311396,
16.9587472215029));
#45737=CARTESIAN_POINT('Ctrl Pts',(-46.4608607449701,-77.0312443703412,
17.5782509142251));
#45738=CARTESIAN_POINT('Ctrl Pts',(-46.320096662837,-75.9317484370967,19.3262399513567));
#45739=CARTESIAN_POINT('Ctrl Pts',(-46.1625627274249,-76.1796390782523,
21.6382820870331));
#45740=CARTESIAN_POINT('Ctrl Pts',(-46.0036976824358,-78.0797604735648,
23.161043382435));
#45741=CARTESIAN_POINT('Ctrl Pts',(-45.875575120692,-79.9539900307661,22.9387587305178));
#45742=CARTESIAN_POINT('Ctrl Pts',(-45.7468693842732,-81.4804681301568,
21.9876429965309));
#45743=CARTESIAN_POINT('Ctrl Pts',(-45.6012748321095,-82.4538170148249,
19.9738849325405));
#45744=CARTESIAN_POINT('Ctrl Pts',(-45.427232277001,-81.2961720285109,17.5655039599756));
#45745=CARTESIAN_POINT('Ctrl Pts',(-45.2739171720439,-79.2134585556205,
16.7610475026127));
#45746=CARTESIAN_POINT('Ctrl Pts',(-45.1417971188088,-77.3459353550754,
17.1811310509974));
#45747=CARTESIAN_POINT('Ctrl Pts',(-45.0090220243129,-76.0316098470263,
18.5974518633508));
#45748=CARTESIAN_POINT('Ctrl Pts',(-44.8755781232189,-75.7405809030124,
20.5124323793354));
#45749=CARTESIAN_POINT('Ctrl Pts',(-44.7415271801667,-76.5852722717957,
22.2695961253322));
#45750=CARTESIAN_POINT('Ctrl Pts',(-44.6180902998809,-78.1379907426961,
23.1657114909166));
#45751=CARTESIAN_POINT('Ctrl Pts',(-44.5054512296313,-79.7434195908802,
23.164944985583));
#45752=CARTESIAN_POINT('Ctrl Pts',(-44.403762511972,-81.0487736199286,22.5375621623098));
#45753=CARTESIAN_POINT('Ctrl Pts',(-44.3187755095097,-81.803927310347,21.5908894911752));
#45754=CARTESIAN_POINT('Ctrl Pts',(-44.2506328752899,-82.1178415065376,
20.6917295984092));
#45755=CARTESIAN_POINT('Ctrl Pts',(-44.182398840638,-82.2256429773631,19.7439125803809));
#45756=CARTESIAN_POINT('Ctrl Pts',(-44.0969322192952,-81.9548232044274,
18.5574476942815));
#45757=CARTESIAN_POINT('Ctrl Pts',(-43.9941104782232,-81.0423485897149,
17.4111483979706));
#45758=CARTESIAN_POINT('Ctrl Pts',(-43.8910383941689,-79.7196940350006,
16.775424120007));
#45759=CARTESIAN_POINT('Ctrl Pts',(-43.7705035162583,-78.002099182994,16.7721223788263));
#45760=CARTESIAN_POINT('Ctrl Pts',(-43.6323887221455,-76.2810481647922,
17.8464747635074));
#45761=CARTESIAN_POINT('Ctrl Pts',(-43.4765588968987,-75.523682339802,20.0119147314719));
#45762=CARTESIAN_POINT('Ctrl Pts',(-43.3203104399421,-76.2814825700852,
22.1798824763609));
#45763=CARTESIAN_POINT('Ctrl Pts',(-43.1636988788655,-78.231183283665,23.4065011857406));
#45764=CARTESIAN_POINT('Ctrl Pts',(-43.0067701275799,-80.5243831967142,
23.1486711821189));
#45765=CARTESIAN_POINT('Ctrl Pts',(-42.8495752732181,-82.1593690722874,
21.5147059359154));
#45766=CARTESIAN_POINT('Ctrl Pts',(-42.692163877366,-82.4189200513296,19.2145330104326));
#45767=CARTESIAN_POINT('Ctrl Pts',(-42.5345870339397,-81.186419702914,17.252341889947));
#45768=CARTESIAN_POINT('Ctrl Pts',(-42.3768955999956,-78.9974076189623,
16.4862760606958));
#45769=CARTESIAN_POINT('Ctrl Pts',(-42.2191420853598,-76.8080962266395,
17.2523251227454));
#45770=CARTESIAN_POINT('Ctrl Pts',(-42.0613769172934,-75.5725384440266,
19.2168395004127));
#45771=CARTESIAN_POINT('Ctrl Pts',(-41.9036550552319,-75.8347814351827,
21.521221016026));
#45772=CARTESIAN_POINT('Ctrl Pts',(-41.7459807111963,-77.472413483267,23.1602525911309));
#45773=CARTESIAN_POINT('Ctrl Pts',(-41.5885306559279,-79.775140966077,23.418780464454));
#45774=CARTESIAN_POINT('Ctrl Pts',(-41.4573307056616,-81.4042927804752,
22.3935048251252));
#45775=CARTESIAN_POINT('Ctrl Pts',(-41.352752520906,-82.115291034017,21.0964799172088));
#45776=CARTESIAN_POINT('Ctrl Pts',(-41.3002494256406,-82.2388355933261,
20.376965989901));
#45777=CARTESIAN_POINT('Ctrl Pts',(-41.2742555650807,-82.2395138211038,
20.0097117288145));
#45778=CARTESIAN_POINT('Ctrl Pts',(-56.4864851473071,-82.244406184525,20.0072137503139));
#45779=CARTESIAN_POINT('Ctrl Pts',(-56.4604905643926,-82.2437279376262,
19.6399492874994));
#45780=CARTESIAN_POINT('Ctrl Pts',(-56.4079575497986,-82.1200108277759,
18.920179834268));
#45781=CARTESIAN_POINT('Ctrl Pts',(-56.3035124971059,-81.4097019511314,
17.6250516252384));
#45782=CARTESIAN_POINT('Ctrl Pts',(-56.1728276535228,-79.7866044363345,
16.6050341645054));
#45783=CARTESIAN_POINT('Ctrl Pts',(-56.0165510858122,-77.5016274012234,
16.8629024989691));
#45784=CARTESIAN_POINT('Ctrl Pts',(-55.860614787854,-75.8832484996987,18.4844935021406));
#45785=CARTESIAN_POINT('Ctrl Pts',(-55.7051693135572,-75.6261404352104,
20.7551980554146));
#45786=CARTESIAN_POINT('Ctrl Pts',(-55.5501938084122,-76.8403636413408,
22.6833784979432));
#45787=CARTESIAN_POINT('Ctrl Pts',(-55.3957875322177,-78.9829092901664,
23.4316620324926));
#45788=CARTESIAN_POINT('Ctrl Pts',(-55.24196914399,-81.1169629091852,22.6834289530792));
#45789=CARTESIAN_POINT('Ctrl Pts',(-55.0887919206184,-82.3135405021836,
20.775923098071));
#45790=CARTESIAN_POINT('Ctrl Pts',(-54.9362912020637,-82.0610299365338,
18.5483313129834));
#45791=CARTESIAN_POINT('Ctrl Pts',(-54.7845085300065,-80.4817755535852,
16.971919870799));
#45792=CARTESIAN_POINT('Ctrl Pts',(-54.6334788977311,-78.2758404106939,
16.725043392695));
#45793=CARTESIAN_POINT('Ctrl Pts',(-54.4832409733484,-76.4057062548225,
17.9022861782441));
#45794=CARTESIAN_POINT('Ctrl Pts',(-54.3587251945716,-75.8050582161101,
19.6298057588485));
#45795=CARTESIAN_POINT('Ctrl Pts',(-54.2595476624192,-76.0424269715925,
21.0072061434664));
#45796=CARTESIAN_POINT('Ctrl Pts',(-54.1853814487781,-76.5470394748316,
21.9218209716504));
#45797=CARTESIAN_POINT('Ctrl Pts',(-54.1114367342337,-77.3244395716799,
22.6148156691908));
#45798=CARTESIAN_POINT('Ctrl Pts',(-54.0131440892721,-78.603436095196,23.1472615029114));
#45799=CARTESIAN_POINT('Ctrl Pts',(-53.89084487041,-80.3887986905675,22.9461526703339));
#45800=CARTESIAN_POINT('Ctrl Pts',(-53.7450274334933,-81.9037455172806,
21.4272424575567));
#45801=CARTESIAN_POINT('Ctrl Pts',(-53.6001717997465,-82.1395116153914,
19.3115740408835));
#45802=CARTESIAN_POINT('Ctrl Pts',(-53.4563014930413,-81.0123159195144,
17.5203471528416));
#45803=CARTESIAN_POINT('Ctrl Pts',(-53.3134327675242,-79.0285454948578,
16.8315743124168));
#45804=CARTESIAN_POINT('Ctrl Pts',(-53.1715865117443,-77.0609306911321,
17.5224129170849));
#45805=CARTESIAN_POINT('Ctrl Pts',(-53.0307741778491,-75.9616236346913,
19.2767822365058));
#45806=CARTESIAN_POINT('Ctrl Pts',(-52.8910084417059,-76.1943323645279,
21.3184594913424));
#45807=CARTESIAN_POINT('Ctrl Pts',(-52.7522984009004,-77.6383558894365,
22.7586903987038));
#45808=CARTESIAN_POINT('Ctrl Pts',(-52.6146512025417,-79.6498424442095,
22.9826023867588));
#45809=CARTESIAN_POINT('Ctrl Pts',(-52.4780713027781,-81.3488556804301,
21.9118659023322));
#45810=CARTESIAN_POINT('Ctrl Pts',(-52.3425607834635,-82.0044406266488,
20.0302316483582));
#45811=CARTESIAN_POINT('Ctrl Pts',(-52.2081191771091,-81.3490236341856,
18.1651768258721));
#45812=CARTESIAN_POINT('Ctrl Pts',(-52.0747434976663,-79.6870258617311,
17.1239828634592));
#45813=CARTESIAN_POINT('Ctrl Pts',(-51.9424282544566,-77.7539297691834,
17.3444231983787));
#45814=CARTESIAN_POINT('Ctrl Pts',(-51.811165533831,-76.3909322893194,18.7110902501839));
#45815=CARTESIAN_POINT('Ctrl Pts',(-51.6809449612247,-76.1790859877837,
20.6141953273701));
#45816=CARTESIAN_POINT('Ctrl Pts',(-51.5517537883029,-77.191947419427,22.2214040979907));
#45817=CARTESIAN_POINT('Ctrl Pts',(-51.4235767560169,-78.9718377059214,
22.841571824978));
#45818=CARTESIAN_POINT('Ctrl Pts',(-51.2963963326679,-80.736261721788,22.22157134421));
#45819=CARTESIAN_POINT('Ctrl Pts',(-51.1701921675022,-81.7215941240923,
20.6488770320107));
#45820=CARTESIAN_POINT('Ctrl Pts',(-51.04494276267,-81.512959740282,18.81889422146));
#45821=CARTESIAN_POINT('Ctrl Pts',(-50.9206221929331,-80.2186251867107,
17.5277455362834));
#45822=CARTESIAN_POINT('Ctrl Pts',(-50.7972074154033,-78.4146002994715,
17.3268756024418));
#45823=CARTESIAN_POINT('Ctrl Pts',(-50.6746620991811,-76.890151497893,18.2872664763635));
#45824=CARTESIAN_POINT('Ctrl Pts',(-50.5529729373044,-76.3000175094954,
19.9778077309354));
#45825=CARTESIAN_POINT('Ctrl Pts',(-50.4320678326896,-76.8908632778512,
21.6540392745149));
#45826=CARTESIAN_POINT('Ctrl Pts',(-50.3119596915113,-78.3872184931367,
22.5923847015876));
#45827=CARTESIAN_POINT('Ctrl Pts',(-50.1925891892237,-80.1314109391504,
22.3940639393699));
#45828=CARTESIAN_POINT('Ctrl Pts',(-50.0739208360292,-81.364151714832,21.1588635538291));
#45829=CARTESIAN_POINT('Ctrl Pts',(-49.9559142964183,-81.5567499157273,
19.4340963825786));
#45830=CARTESIAN_POINT('Ctrl Pts',(-49.8385286442904,-80.6369710758383,
17.9731922877536));
#45831=CARTESIAN_POINT('Ctrl Pts',(-49.7217215196508,-79.0147721014308,
17.4069911561483));
#45832=CARTESIAN_POINT('Ctrl Pts',(-49.6054475819526,-77.4013710218261,
17.9732338854577));
#45833=CARTESIAN_POINT('Ctrl Pts',(-49.4896640315131,-76.4954328808651,
19.4150710735183));
#45834=CARTESIAN_POINT('Ctrl Pts',(-49.3743185623355,-76.6880905927546,
21.1019689204466));
#45835=CARTESIAN_POINT('Ctrl Pts',(-49.2593775009166,-77.8799327853689,
22.293670540459));
#45836=CARTESIAN_POINT('Ctrl Pts',(-49.1320281323078,-79.7504014899488,
22.5091749028563));
#45837=CARTESIAN_POINT('Ctrl Pts',(-49.0177356327972,-81.1156454492951,
21.4212181211584));
#45838=CARTESIAN_POINT('Ctrl Pts',(-48.9226956524205,-81.4083679794129,
20.0913953086005));
#45839=CARTESIAN_POINT('Ctrl Pts',(-48.8594012746119,-81.2602898532879,
19.2152150535946));
#45840=CARTESIAN_POINT('Ctrl Pts',(-48.7834990124813,-80.743690351567,18.2765978302752));
#45841=CARTESIAN_POINT('Ctrl Pts',(-48.6887409077433,-79.5658058177838,
17.5354801724578));
#45842=CARTESIAN_POINT('Ctrl Pts',(-48.5751083143484,-77.9040028995463,
17.7226483218797));
#45843=CARTESIAN_POINT('Ctrl Pts',(-48.4615222697365,-76.7233535485495,
18.9039803371791));
#45844=CARTESIAN_POINT('Ctrl Pts',(-48.3479226073069,-76.5359862699538,
20.5641246869877));
#45845=CARTESIAN_POINT('Ctrl Pts',(-48.2342619825293,-77.4252520533088,
21.9796151711007));
#45846=CARTESIAN_POINT('Ctrl Pts',(-48.1204872312989,-79.004419957339,22.5325711539792));
#45847=CARTESIAN_POINT('Ctrl Pts',(-48.0065478245435,-80.5861911385054,
21.9795902880699));
#45848=CARTESIAN_POINT('Ctrl Pts',(-47.8923923883356,-81.4798322178271,
20.5584387533152));
#45849=CARTESIAN_POINT('Ctrl Pts',(-47.7779709658212,-81.2921160797888,
18.8862371910536));
#45850=CARTESIAN_POINT('Ctrl Pts',(-47.6632337755331,-80.0995238430424,
17.692561192887));
#45851=CARTESIAN_POINT('Ctrl Pts',(-47.5481326792351,-78.4175602791118,
17.5020376251063));
#45852=CARTESIAN_POINT('Ctrl Pts',(-47.4326186963439,-76.9784793998031,
18.4050558861712));
#45853=CARTESIAN_POINT('Ctrl Pts',(-47.3166472249995,-76.4140883364296,
20.0141330991597));
#45854=CARTESIAN_POINT('Ctrl Pts',(-47.2001668836196,-76.9781174597249,
21.6320696043394));
#45855=CARTESIAN_POINT('Ctrl Pts',(-47.102648679663,-78.1922506890227,22.3947478975612));
#45856=CARTESIAN_POINT('Ctrl Pts',(-47.0243227633107,-79.2934240076467,
22.4539599055311));
#45857=CARTESIAN_POINT('Ctrl Pts',(-46.9457927494229,-80.3599158358455,
22.1509640171201));
#45858=CARTESIAN_POINT('Ctrl Pts',(-46.8603764354211,-81.2434007966227,
21.2659119848418));
#45859=CARTESIAN_POINT('Ctrl Pts',(-46.741537508699,-81.6262476288813,19.6101004829355));
#45860=CARTESIAN_POINT('Ctrl Pts',(-46.6568637398311,-81.0760751285665,
18.442619615091));
#45861=CARTESIAN_POINT('Ctrl Pts',(-46.5934814534038,-80.3608237881132,
17.9244206785242));
#45862=CARTESIAN_POINT('Ctrl Pts',(-46.5534170582025,-79.8858191183262,
17.634331035083));
#45863=CARTESIAN_POINT('Ctrl Pts',(-46.4780913513627,-78.8402806753656,
17.3620372339516));
#45864=CARTESIAN_POINT('Ctrl Pts',(-46.3669961151747,-77.2955789649705,
17.8997405417894));
#45865=CARTESIAN_POINT('Ctrl Pts',(-46.244957124377,-76.3424755180359,19.4152946981647));
#45866=CARTESIAN_POINT('Ctrl Pts',(-46.1084247765798,-76.557423872972,21.4190561415109));
#45867=CARTESIAN_POINT('Ctrl Pts',(-45.9707329691292,-78.2041668358601,
22.7389476836005));
#45868=CARTESIAN_POINT('Ctrl Pts',(-45.8596256684999,-79.8294782506187,
22.5463669763199));
#45869=CARTESIAN_POINT('Ctrl Pts',(-45.7479534244289,-81.1538676554818,
21.7211828863017));
#45870=CARTESIAN_POINT('Ctrl Pts',(-45.6215284524728,-81.9995992769805,
19.9729588911492));
#45871=CARTESIAN_POINT('Ctrl Pts',(-45.4701335388581,-80.9935962179004,
17.8777328348881));
#45872=CARTESIAN_POINT('Ctrl Pts',(-45.3364999414446,-79.1787132506225,
17.1761128984294));
#45873=CARTESIAN_POINT('Ctrl Pts',(-45.2211494416365,-77.5482952105881,
17.5424430554541));
#45874=CARTESIAN_POINT('Ctrl Pts',(-45.1049770492795,-76.3982092929863,
18.7809644843786));
#45875=CARTESIAN_POINT('Ctrl Pts',(-44.9879827710476,-76.1425303947159,
20.4596334384395));
#45876=CARTESIAN_POINT('Ctrl Pts',(-44.8701487351934,-76.8842395494568,
22.0040483067461));
#45877=CARTESIAN_POINT('Ctrl Pts',(-44.7613669966606,-78.2519997258415,
22.7941158256609));
#45878=CARTESIAN_POINT('Ctrl Pts',(-44.6618625928431,-79.6699579690279,
22.7937774228697));
#45879=CARTESIAN_POINT('Ctrl Pts',(-44.5718347215401,-80.8255497018144,
22.238718741254));
#45880=CARTESIAN_POINT('Ctrl Pts',(-44.4964128977026,-81.4957557167802,
21.3989808934452));
#45881=CARTESIAN_POINT('Ctrl Pts',(-44.4358432233994,-81.7748194347551,
20.5998204980552));
#45882=CARTESIAN_POINT('Ctrl Pts',(-44.3751132847541,-81.8708038494031,
19.756384583514));
#45883=CARTESIAN_POINT('Ctrl Pts',(-44.2989055206723,-81.6296514379495,
18.6985105124891));
#45884=CARTESIAN_POINT('Ctrl Pts',(-44.2069805398381,-80.8143272807318,
17.6736395231787));
#45885=CARTESIAN_POINT('Ctrl Pts',(-44.1145834563323,-79.6290317450135,
17.1034965275683));
#45886=CARTESIAN_POINT('Ctrl Pts',(-44.0062428609622,-78.0854298017345,
17.1000390392989));
#45887=CARTESIAN_POINT('Ctrl Pts',(-43.8816346938952,-76.5325285282763,
18.067897428711));
#45888=CARTESIAN_POINT('Ctrl Pts',(-43.7403998945461,-75.8448247700219,
20.0291730208815));
#45889=CARTESIAN_POINT('Ctrl Pts',(-43.5981411706491,-76.5329789950227,
22.002878837303));
#45890=CARTESIAN_POINT('Ctrl Pts',(-43.4548672770674,-78.3150063887284,
23.126063236142));
#45891=CARTESIAN_POINT('Ctrl Pts',(-43.3105981900307,-80.4226136408398,
22.8909180049375));
#45892=CARTESIAN_POINT('Ctrl Pts',(-43.1653527245271,-81.9340396600559,
21.3830760708777));
#45893=CARTESIAN_POINT('Ctrl Pts',(-43.0191522761607,-82.17692827644,19.2478221178909));
#45894=CARTESIAN_POINT('Ctrl Pts',(-42.8720229653157,-81.0283119211314,
17.4154508680147));
#45895=CARTESIAN_POINT('Ctrl Pts',(-42.72398589125,-78.9749522023299,16.6947394827832));
#45896=CARTESIAN_POINT('Ctrl Pts',(-42.5750811952544,-76.9086922943806,
17.4156052640251));
#45897=CARTESIAN_POINT('Ctrl Pts',(-42.4253130086118,-75.7347412322853,
19.2784528703265));
#45898=CARTESIAN_POINT('Ctrl Pts',(-42.2747717246015,-75.9829440186284,
21.4774728284354));
#45899=CARTESIAN_POINT('Ctrl Pts',(-42.1234329434898,-77.5530085323627,
23.0518956352805));
#45900=CARTESIAN_POINT('Ctrl Pts',(-41.9714093758298,-79.7755362218638,
23.3034733604654));
#45901=CARTESIAN_POINT('Ctrl Pts',(-41.8440182230729,-81.3582430385855,
22.3099349163572));
#45902=CARTESIAN_POINT('Ctrl Pts',(-41.7419838188056,-82.0522110516402,
21.0447471654702));
#45903=CARTESIAN_POINT('Ctrl Pts',(-41.6906401481783,-82.173201565315,20.3413153591936));
#45904=CARTESIAN_POINT('Ctrl Pts',(-41.6652025102081,-82.1738652802192,
19.9819196890115));
#45905=CARTESIAN_POINT('Ctrl Pts',(-56.8752592603261,-82.1647273768201,
19.9798438846464));
#45906=CARTESIAN_POINT('Ctrl Pts',(-56.849820483618,-82.1640636319366,19.6204321297793));
#45907=CARTESIAN_POINT('Ctrl Pts',(-56.7985225143976,-82.0433810770499,
18.9174518831814));
#45908=CARTESIAN_POINT('Ctrl Pts',(-56.6961514981416,-81.3476586777129,
17.6477773877481));
#45909=CARTESIAN_POINT('Ctrl Pts',(-56.5675242515753,-79.750819824018,16.6421258544651));
#45910=CARTESIAN_POINT('Ctrl Pts',(-56.4127777672657,-77.4877184491089,
16.8951938814764));
#45911=CARTESIAN_POINT('Ctrl Pts',(-56.2574474727138,-75.8738250468064,
18.5092015929225));
#45912=CARTESIAN_POINT('Ctrl Pts',(-56.1016864083364,-75.6139448078687,
20.7846026649799));
#45913=CARTESIAN_POINT('Ctrl Pts',(-55.9454946697642,-76.8362502840664,
22.7298037295438));
#45914=CARTESIAN_POINT('Ctrl Pts',(-55.7889342465819,-79.0084823141423,
23.4908597602889));
#45915=CARTESIAN_POINT('Ctrl Pts',(-55.6320475439178,-81.1864409267459,
22.7296922749762));
#45916=CARTESIAN_POINT('Ctrl Pts',(-55.4748870696447,-82.4163634726471,
20.7734068870129));
#45917=CARTESIAN_POINT('Ctrl Pts',(-55.3175017283399,-82.1580193500458,
18.4737774574898));
#45918=CARTESIAN_POINT('Ctrl Pts',(-55.1599423980537,-80.5200128949239,
16.8354996081942));
#45919=CARTESIAN_POINT('Ctrl Pts',(-55.0022599601601,-78.2168457221201,
16.5754940197918));
#45920=CARTESIAN_POINT('Ctrl Pts',(-54.8445051279008,-76.2517211817873,
17.8098895741297));
#45921=CARTESIAN_POINT('Ctrl Pts',(-54.7130265903422,-75.6157428815775,
19.6337203952621));
#45922=CARTESIAN_POINT('Ctrl Pts',(-54.6078575942801,-75.8671226247866,
21.0945269420162));
#45923=CARTESIAN_POINT('Ctrl Pts',(-54.5289952123769,-76.4034892139563,
22.0671944258025));
#45924=CARTESIAN_POINT('Ctrl Pts',(-54.45015348062,-77.2322557766833,22.8063001739345));
#45925=CARTESIAN_POINT('Ctrl Pts',(-54.3450673578701,-78.5994774058443,
23.3758588243804));
#45926=CARTESIAN_POINT('Ctrl Pts',(-54.2137934297236,-80.5160729256162,
23.1616447909686));
#45927=CARTESIAN_POINT('Ctrl Pts',(-54.0564493591351,-82.1522391523417,
21.5241073076164));
#45928=CARTESIAN_POINT('Ctrl Pts',(-53.8993416236473,-82.4098810996251,
19.2296924343533));
#45929=CARTESIAN_POINT('Ctrl Pts',(-53.7425168108729,-81.182881687469,17.2762363265303));
#45930=CARTESIAN_POINT('Ctrl Pts',(-53.5860317510178,-79.0106245714821,
16.5200699813797));
#45931=CARTESIAN_POINT('Ctrl Pts',(-53.4299252093456,-76.8447807469938,
17.278626424945));
#45932=CARTESIAN_POINT('Ctrl Pts',(-53.2742504725809,-75.6280966857697,
19.2170863781129));
#45933=CARTESIAN_POINT('Ctrl Pts',(-53.119053328739,-75.8848398803048,21.4841287570035));
#45934=CARTESIAN_POINT('Ctrl Pts',(-52.9643793906807,-77.4937457201632,
23.0910239089316));
#45935=CARTESIAN_POINT('Ctrl Pts',(-52.8102726712708,-79.7452709481134,
23.3431554210652));
#45936=CARTESIAN_POINT('Ctrl Pts',(-52.6567761139084,-81.6551584863882,
22.1411843335501));
#45937=CARTESIAN_POINT('Ctrl Pts',(-52.503931172354,-82.3957109528423,20.0196751705757));
#45938=CARTESIAN_POINT('Ctrl Pts',(-52.351778100954,-81.6552494754696,17.9089395610088));
#45939=CARTESIAN_POINT('Ctrl Pts',(-52.2003554700587,-79.769380504285,16.7261729823972));
#45940=CARTESIAN_POINT('Ctrl Pts',(-52.0496999603813,-77.5687465705001,
16.9760925231193));
#45941=CARTESIAN_POINT('Ctrl Pts',(-51.8998463388462,-76.012452612391,18.5352706051618));
#45942=CARTESIAN_POINT('Ctrl Pts',(-51.7508275550648,-75.7692773993649,
20.7124125039816));
#45943=CARTESIAN_POINT('Ctrl Pts',(-51.6026745746877,-76.9298555111948,
22.5553551303563));
#45944=CARTESIAN_POINT('Ctrl Pts',(-51.4554165147952,-78.9738720391516,
23.268189846291));
#45945=CARTESIAN_POINT('Ctrl Pts',(-51.3090803638474,-81.0035379035248,
22.5555024258079));
#45946=CARTESIAN_POINT('Ctrl Pts',(-51.1636912979732,-82.1385729582828,
20.7445599295758));
#45947=CARTESIAN_POINT('Ctrl Pts',(-51.0192712722321,-81.8983414763417,
18.6352378679758));
#45948=CARTESIAN_POINT('Ctrl Pts',(-50.8758418420892,-80.4057039065717,
17.1460946436865));
#45949=CARTESIAN_POINT('Ctrl Pts',(-50.7334180548278,-78.3246929559324,
16.9143845079462));
#45950=CARTESIAN_POINT('Ctrl Pts',(-50.59202195101,-76.5664296105997,18.0221939935554));
#45951=CARTESIAN_POINT('Ctrl Pts',(-50.4516523555111,-75.8863075302345,
19.9712950019085));
#45952=CARTESIAN_POINT('Ctrl Pts',(-50.3123526988948,-76.567215386836,21.9020278716489));
#45953=CARTESIAN_POINT('Ctrl Pts',(-50.1740919754148,-78.2891689544036,
22.9812616932865));
#45954=CARTESIAN_POINT('Ctrl Pts',(-50.0368949024821,-80.2928434997237,
22.7528430998679));
#45955=CARTESIAN_POINT('Ctrl Pts',(-49.9007628172212,-81.7058263131614,
21.3360544397924));
#45956=CARTESIAN_POINT('Ctrl Pts',(-49.7656971633282,-81.9253505848977,
19.3628482967946));
#45957=CARTESIAN_POINT('Ctrl Pts',(-49.6316962630047,-80.875132507514,17.696518464657));
#45958=CARTESIAN_POINT('Ctrl Pts',(-49.4987557206264,-79.0295187448053,
17.0534789042926));
#45959=CARTESIAN_POINT('Ctrl Pts',(-49.3668698109708,-77.2008650160025,
17.6965257519911));
#45960=CARTESIAN_POINT('Ctrl Pts',(-49.2360272361897,-76.1788139886115,
19.3257142409972));
#45961=CARTESIAN_POINT('Ctrl Pts',(-49.1062212407889,-76.3969375716729,
21.2228970450781));
#45962=CARTESIAN_POINT('Ctrl Pts',(-48.9774270334425,-77.7326214921823,
22.5564587298384));
#45963=CARTESIAN_POINT('Ctrl Pts',(-48.8354545460198,-79.8173749253273,
22.7945675099833));
#45964=CARTESIAN_POINT('Ctrl Pts',(-48.7088470418068,-81.3278881573385,
21.5873043990266));
#45965=CARTESIAN_POINT('Ctrl Pts',(-48.6041290543196,-81.649373826429,20.1224911974117));
#45966=CARTESIAN_POINT('Ctrl Pts',(-48.534620354474,-81.4866810139768,19.1606355190012));
#45967=CARTESIAN_POINT('Ctrl Pts',(-48.4515237794181,-80.9208898398131,
18.1333862032429));
#45968=CARTESIAN_POINT('Ctrl Pts',(-48.3482038580319,-79.6366194811744,
17.3271167141711));
#45969=CARTESIAN_POINT('Ctrl Pts',(-48.2251202545579,-77.837643114993,17.5317437994423));
#45970=CARTESIAN_POINT('Ctrl Pts',(-48.1028920056514,-76.5693020567696,
18.8036614028563));
#45971=CARTESIAN_POINT('Ctrl Pts',(-47.9814941498671,-76.3712437839294,
20.5771187760201));
#45972=CARTESIAN_POINT('Ctrl Pts',(-47.8608902646939,-77.3161881337434,
22.0771677966622));
#45973=CARTESIAN_POINT('Ctrl Pts',(-47.7410462421363,-78.9795365673136,
22.6572563470884));
#45974=CARTESIAN_POINT('Ctrl Pts',(-47.621924133136,-80.6317614090933,22.0772596720609));
#45975=CARTESIAN_POINT('Ctrl Pts',(-47.5034851640459,-81.5566082922497,
20.6022109593297));
#45976=CARTESIAN_POINT('Ctrl Pts',(-47.3856887008372,-81.3611652480675,
18.8816656058404));
#45977=CARTESIAN_POINT('Ctrl Pts',(-47.2684930379886,-80.1418965970207,
17.6645313415393));
#45978=CARTESIAN_POINT('Ctrl Pts',(-47.1518546779662,-78.4378987159531,
17.4738303532817));
#45979=CARTESIAN_POINT('Ctrl Pts',(-47.035729680131,-76.9929991848448,18.3832266388075));
#45980=CARTESIAN_POINT('Ctrl Pts',(-46.9200707020022,-76.4325170788587,
19.9880981973879));
#45981=CARTESIAN_POINT('Ctrl Pts',(-46.8048338212136,-76.9925383820305,
21.5874694958995));
#45982=CARTESIAN_POINT('Ctrl Pts',(-46.7091081845317,-78.1847792549115,
22.334195828462));
#45983=CARTESIAN_POINT('Ctrl Pts',(-46.6326982675346,-79.2587887541768,
22.3916117914154));
#45984=CARTESIAN_POINT('Ctrl Pts',(-46.5563871527435,-80.2949437910353,
22.0967756284929));
#45985=CARTESIAN_POINT('Ctrl Pts',(-46.4738638160743,-81.1473553294667,
21.2409040031375));
#45986=CARTESIAN_POINT('Ctrl Pts',(-46.3597902157357,-81.513659560961,19.6513176505422));
#45987=CARTESIAN_POINT('Ctrl Pts',(-46.2791218208211,-80.9873379664293,
18.539972764432));
#45988=CARTESIAN_POINT('Ctrl Pts',(-46.2190639506903,-80.3096902111283,
18.0491241809696));
#45989=CARTESIAN_POINT('Ctrl Pts',(-46.1811383237244,-79.8600373014878,
17.7745096412059));
#45990=CARTESIAN_POINT('Ctrl Pts',(-46.110055836894,-78.8732147621218,17.5182574519196));
#45991=CARTESIAN_POINT('Ctrl Pts',(-46.0058525452064,-77.4252814529119,
18.0242139470201));
#45992=CARTESIAN_POINT('Ctrl Pts',(-45.8922026265434,-76.539210510756,19.4365393731754));
#45993=CARTESIAN_POINT('Ctrl Pts',(-45.7658834584667,-76.7403618945056,
21.2900242272622));
#45994=CARTESIAN_POINT('Ctrl Pts',(-45.6394596654201,-78.254383737651,22.4991687889416));
#45995=CARTESIAN_POINT('Ctrl Pts',(-45.5381619454123,-79.735719356395,22.3220960440989));
#45996=CARTESIAN_POINT('Ctrl Pts',(-45.4367445560468,-80.9384968216192,
21.5724769602265));
#45997=CARTESIAN_POINT('Ctrl Pts',(-45.3224673093312,-81.7004093138281,
19.9911131458827));
#45998=CARTESIAN_POINT('Ctrl Pts',(-45.1865750493327,-80.7945960871807,
18.1116772564183));
#45999=CARTESIAN_POINT('Ctrl Pts',(-45.067267809229,-79.1739536659866,17.4864162444988));
#46000=CARTESIAN_POINT('Ctrl Pts',(-44.9646874949972,-77.7240469630762,
17.8129469503058));
#46001=CARTESIAN_POINT('Ctrl Pts',(-44.8617690078026,-76.7056236007332,
18.910928891785));
#46002=CARTESIAN_POINT('Ctrl Pts',(-44.7584641908549,-76.480539316094,20.3933934365883));
#46003=CARTESIAN_POINT('Ctrl Pts',(-44.6547587194653,-77.1340685669796,
21.7526435901753));
#46004=CARTESIAN_POINT('Ctrl Pts',(-44.5592880723631,-78.3349402974165,
22.4457038177027));
#46005=CARTESIAN_POINT('Ctrl Pts',(-44.4721509081512,-79.576854086323,22.4451636374686));
#46006=CARTESIAN_POINT('Ctrl Pts',(-44.3934483384747,-80.5871463859038,
21.9596778440093));
#46007=CARTESIAN_POINT('Ctrl Pts',(-44.3276243811037,-81.1720812201823,
21.226542345069));
#46008=CARTESIAN_POINT('Ctrl Pts',(-44.274808294589,-81.4154125231196,20.5296318079551));
#46009=CARTESIAN_POINT('Ctrl Pts',(-44.2218917840583,-81.4990363304231,
19.7946015755715));
#46010=CARTESIAN_POINT('Ctrl Pts',(-44.1555489539339,-81.2889560814031,
18.8735938810967));
#46011=CARTESIAN_POINT('Ctrl Pts',(-44.0756146123583,-80.5797685906883,
17.9823336840274));
#46012=CARTESIAN_POINT('Ctrl Pts',(-43.9953446131058,-79.5498136667998,
17.4870332901371));
#46013=CARTESIAN_POINT('Ctrl Pts',(-43.9012877875629,-78.2095611820704,
17.4841349207429));
#46014=CARTESIAN_POINT('Ctrl Pts',(-43.7932102496733,-76.8623578132868,
18.3240159758579));
#46015=CARTESIAN_POINT('Ctrl Pts',(-43.6707955883791,-76.2661491824651,
20.024684650845));
#46016=CARTESIAN_POINT('Ctrl Pts',(-43.5475096262792,-76.8627315678271,
21.7357943752776));
#46017=CARTESIAN_POINT('Ctrl Pts',(-43.4233292629246,-78.4078293249966,
22.7097747478266));
#46018=CARTESIAN_POINT('Ctrl Pts',(-43.2982253749316,-80.2361879343779,
22.5059992916388));
#46019=CARTESIAN_POINT('Ctrl Pts',(-43.1721744015948,-81.5486128680076,
21.1971050757497));
#46020=CARTESIAN_POINT('Ctrl Pts',(-43.0451541452452,-81.7600970908285,
19.3412274997668));
#46021=CARTESIAN_POINT('Ctrl Pts',(-42.9171435660302,-80.7606861815771,
17.7460023752414));
#46022=CARTESIAN_POINT('Ctrl Pts',(-42.7881277014792,-78.9703896149554,
17.1170309454072));
#46023=CARTESIAN_POINT('Ctrl Pts',(-42.6580847566778,-77.1647690829171,
17.7461949009107));
#46024=CARTESIAN_POINT('Ctrl Pts',(-42.5270162280679,-76.1358663680163,
19.3771917235364));
#46025=CARTESIAN_POINT('Ctrl Pts',(-42.3948798007065,-76.3528431108269,
21.3079390832326));
#46026=CARTESIAN_POINT('Ctrl Pts',(-42.2616851225389,-77.7343788134307,
22.6951866504985));
#46027=CARTESIAN_POINT('Ctrl Pts',(-42.1274243440262,-79.6971490024854,
22.9179776480344));
#46028=CARTESIAN_POINT('Ctrl Pts',(-42.014670143851,-81.0996489509398,22.0396067694999));
#46029=CARTESIAN_POINT('Ctrl Pts',(-41.9239057210112,-81.7167415335571,
20.9138412402982));
#46030=CARTESIAN_POINT('Ctrl Pts',(-41.8783332471008,-81.8242677093701,
20.2893946603941));
#46031=CARTESIAN_POINT('Ctrl Pts',(-41.8555711999267,-81.8248616131743,
19.9678010749981));
#46032=CARTESIAN_POINT('Ctrl Pts',(-56.9957437894396,-81.9300461410118,
19.971749517882));
#46033=CARTESIAN_POINT('Ctrl Pts',(-56.9720878172747,-81.9294289128066,
19.6375261168725));
#46034=CARTESIAN_POINT('Ctrl Pts',(-56.9246413144741,-81.8177633897353,
18.9873413433035));
#46035=CARTESIAN_POINT('Ctrl Pts',(-56.8295978260608,-81.172295314983,17.8084446380066));
#46036=CARTESIAN_POINT('Ctrl Pts',(-56.7100918560198,-79.6886388558644,
16.8738035209148));
#46037=CARTESIAN_POINT('Ctrl Pts',(-56.5658678859323,-77.5795917259262,
17.1083394260631));
#46038=CARTESIAN_POINT('Ctrl Pts',(-56.4207376045591,-76.0708561854358,
18.615883976467));
#46039=CARTESIAN_POINT('Ctrl Pts',(-56.2747745518288,-75.8262259255696,
20.747841123805));
#46040=CARTESIAN_POINT('Ctrl Pts',(-56.1279819285444,-76.973974321702,22.5766823449522));
#46041=CARTESIAN_POINT('Ctrl Pts',(-55.9803900390286,-79.0213695189193,
23.2952423817352));
#46042=CARTESIAN_POINT('Ctrl Pts',(-55.832025105169,-81.0814642752292,22.5765597878218));
#46043=CARTESIAN_POINT('Ctrl Pts',(-55.682917594715,-82.2494586027885,20.7210911241734));
#46044=CARTESIAN_POINT('Ctrl Pts',(-55.5330991431064,-82.0047795818836,
18.5317276122314));
#46045=CARTESIAN_POINT('Ctrl Pts',(-55.3826016766804,-80.4409685466629,
16.9658035999932));
#46046=CARTESIAN_POINT('Ctrl Pts',(-55.2314623577778,-78.233256374022,16.715215318237));
#46047=CARTESIAN_POINT('Ctrl Pts',(-55.0797112113575,-76.3419404793175,
17.9015819532036));
#46048=CARTESIAN_POINT('Ctrl Pts',(-54.9527851585667,-75.7267686910698,
19.6622433798203));
#46049=CARTESIAN_POINT('Ctrl Pts',(-54.8509618033697,-75.9699335874656,
21.0767733443915));
#46050=CARTESIAN_POINT('Ctrl Pts',(-54.7744678880113,-76.4900881076259,
22.0203926993287));
#46051=CARTESIAN_POINT('Ctrl Pts',(-54.6978511000632,-77.2954494492304,
22.7388596335825));
#46052=CARTESIAN_POINT('Ctrl Pts',(-54.5955361546865,-78.626606066821,23.2936701301925));
#46053=CARTESIAN_POINT('Ctrl Pts',(-54.4673860500643,-80.4982210477155,
23.0857086092053));
#46054=CARTESIAN_POINT('Ctrl Pts',(-54.3131881300118,-82.1031550636772,
21.4816044105671));
#46055=CARTESIAN_POINT('Ctrl Pts',(-54.1586231171422,-82.3581618493084,
19.2239374375668));
#46056=CARTESIAN_POINT('Ctrl Pts',(-54.003750320265,-81.1473256829115,17.2932949130607));
#46057=CARTESIAN_POINT('Ctrl Pts',(-53.8485668683044,-78.9932739136752,
16.5418724180722));
#46058=CARTESIAN_POINT('Ctrl Pts',(-53.6931792503979,-76.836159548567,17.2957199364878));
#46059=CARTESIAN_POINT('Ctrl Pts',(-53.5376043604849,-75.6185266026793,
19.2327575977176));
#46060=CARTESIAN_POINT('Ctrl Pts',(-53.3818919303312,-75.874664526356,21.5083040823326));
#46061=CARTESIAN_POINT('Ctrl Pts',(-53.2260876155861,-77.4948156925005,
23.1286340455996));
#46062=CARTESIAN_POINT('Ctrl Pts',(-53.0702387399007,-79.7724813964587,
23.3852583119079));
#46063=CARTESIAN_POINT('Ctrl Pts',(-52.9143921490795,-81.713192088748,22.1657213517522));
#46064=CARTESIAN_POINT('Ctrl Pts',(-52.7585949551581,-82.46980977515,20.0028714955218));
#46065=CARTESIAN_POINT('Ctrl Pts',(-52.602894351696,-81.7132156482904,17.8415191196344));
#46066=CARTESIAN_POINT('Ctrl Pts',(-52.44733732548,-79.7758359678184,16.6246532457464));
#46067=CARTESIAN_POINT('Ctrl Pts',(-52.2919702655199,-77.5052173825921,
16.8810081968058));
#46068=CARTESIAN_POINT('Ctrl Pts',(-52.1368389777891,-75.8923408919337,
18.4947736518063));
#46069=CARTESIAN_POINT('Ctrl Pts',(-51.9819887183747,-75.6380824394838,
20.7579855405843));
#46070=CARTESIAN_POINT('Ctrl Pts',(-51.8274641395511,-76.8479253296823,
22.6818497208179));
#46071=CARTESIAN_POINT('Ctrl Pts',(-51.6733091246767,-78.9882310561524,
23.4297519524038));
#46072=CARTESIAN_POINT('Ctrl Pts',(-51.5195672315392,-81.1221058384755,
22.6819274088254));
#46073=CARTESIAN_POINT('Ctrl Pts',(-51.3662803627253,-82.3205231170056,
20.7723832742744));
#46074=CARTESIAN_POINT('Ctrl Pts',(-51.2134906309633,-82.067536758452,18.5395357722326));
#46075=CARTESIAN_POINT('Ctrl Pts',(-51.0612355077352,-80.4831665052501,
16.9570782370458));
#46076=CARTESIAN_POINT('Ctrl Pts',(-50.9095589525399,-78.2658943169774,
16.7089499791194));
#46077=CARTESIAN_POINT('Ctrl Pts',(-50.7584862188345,-76.3858276880046,
17.8921278081452));
#46078=CARTESIAN_POINT('Ctrl Pts',(-50.6080801931949,-75.6555081289303,
19.9815434149077));
#46079=CARTESIAN_POINT('Ctrl Pts',(-50.4583150157542,-76.3867863899377,
22.0582342796407));
#46080=CARTESIAN_POINT('Ctrl Pts',(-50.3092957305894,-78.2431770442968,
23.2229562447285));
#46081=CARTESIAN_POINT('Ctrl Pts',(-50.1610199298396,-80.4098753634881,
22.97691940353));
#46082=CARTESIAN_POINT('Ctrl Pts',(-50.0135202964699,-81.9422769935299,
21.4416476757106));
#46083=CARTESIAN_POINT('Ctrl Pts',(-49.8668235155934,-82.1816514238649,
19.2974799656789));
#46084=CARTESIAN_POINT('Ctrl Pts',(-49.7209554829974,-81.038468925659,17.4822050937547));
#46085=CARTESIAN_POINT('Ctrl Pts',(-49.5759405288341,-79.0243729605365,
16.7796992026714));
#46086=CARTESIAN_POINT('Ctrl Pts',(-49.4317994982005,-77.0245243396262,
17.4822411066595));
#46087=CARTESIAN_POINT('Ctrl Pts',(-49.2885552045132,-75.9044564152709,
19.2664840098316));
#46088=CARTESIAN_POINT('Ctrl Pts',(-49.1462191456824,-76.1432283129171,
21.3478786801514));
#46089=CARTESIAN_POINT('Ctrl Pts',(-49.0048212758934,-77.6101485651985,
22.813088681206));
#46090=CARTESIAN_POINT('Ctrl Pts',(-48.8487356825073,-79.9029287381131,
23.075400288994));
#46091=CARTESIAN_POINT('Ctrl Pts',(-48.7093468797834,-81.5663232868859,
21.746536954466));
#46092=CARTESIAN_POINT('Ctrl Pts',(-48.5940037608329,-81.9206064075348,
20.1326883641399));
#46093=CARTESIAN_POINT('Ctrl Pts',(-48.5174232874096,-81.741320931239,19.0727142447915));
#46094=CARTESIAN_POINT('Ctrl Pts',(-48.4258458131364,-81.1177007039368,
17.9404149812607));
#46095=CARTESIAN_POINT('Ctrl Pts',(-48.3120022564393,-79.7019158587733,
17.0515806518557));
#46096=CARTESIAN_POINT('Ctrl Pts',(-48.1763524335297,-77.7185967734674,
17.2772440131571));
#46097=CARTESIAN_POINT('Ctrl Pts',(-48.0416796916409,-76.320687388509,18.6793406519538));
#46098=CARTESIAN_POINT('Ctrl Pts',(-47.9079753617284,-76.1027042059027,
20.6332804614806));
#46099=CARTESIAN_POINT('Ctrl Pts',(-47.7752376830806,-77.1433202924972,
22.2846464781002));
#46100=CARTESIAN_POINT('Ctrl Pts',(-47.6434585171334,-78.972990052141,22.9223505322969));
#46101=CARTESIAN_POINT('Ctrl Pts',(-47.5126292328511,-80.7879405549371,
22.2847608704201));
#46102=CARTESIAN_POINT('Ctrl Pts',(-47.3827381427943,-81.8020110648646,
20.6664188218262));
#46103=CARTESIAN_POINT('Ctrl Pts',(-47.2537717088521,-81.5873850261729,
18.7823941819149));
#46104=CARTESIAN_POINT('Ctrl Pts',(-47.1257142248705,-80.2543820614397,
17.452698786342));
#46105=CARTESIAN_POINT('Ctrl Pts',(-46.9985476751261,-78.3961966011715,
17.2455162857473));
#46106=CARTESIAN_POINT('Ctrl Pts',(-46.8722525809472,-76.8250061389063,
18.2353999825299));
#46107=CARTESIAN_POINT('Ctrl Pts',(-46.7468058450621,-76.2178906475949,
19.976571843654));
#46108=CARTESIAN_POINT('Ctrl Pts',(-46.6221857531722,-76.8245123203334,
21.7059764500968));
#46109=CARTESIAN_POINT('Ctrl Pts',(-46.5189980363482,-78.1102171954823,
22.5102013483286));
#46110=CARTESIAN_POINT('Ctrl Pts',(-46.4368404123711,-79.264997126938,22.5717632225066));
#46111=CARTESIAN_POINT('Ctrl Pts',(-46.3549353191113,-80.3771028622425,
22.2550763842303));
#46112=CARTESIAN_POINT('Ctrl Pts',(-46.2666032496695,-81.2889540598721,
21.3384880705053));
#46113=CARTESIAN_POINT('Ctrl Pts',(-46.144898284069,-81.6791110052382,19.6423622368182));
#46114=CARTESIAN_POINT('Ctrl Pts',(-46.0591734169203,-81.1185247625248,
18.4619314156135));
#46115=CARTESIAN_POINT('Ctrl Pts',(-45.9955525435571,-80.4007191749686,
17.9420736696449));
#46116=CARTESIAN_POINT('Ctrl Pts',(-45.9553997199636,-79.9246659480749,
17.6513316937921));
#46117=CARTESIAN_POINT('Ctrl Pts',(-45.8802818055934,-78.8817219091746,
17.3809925802952));
#46118=CARTESIAN_POINT('Ctrl Pts',(-45.7705555090585,-77.3580643432502,
17.9148058039039));
#46119=CARTESIAN_POINT('Ctrl Pts',(-45.651478880851,-76.4308117831266,19.3952080057491));
#46120=CARTESIAN_POINT('Ctrl Pts',(-45.51970485512,-76.642423188315,21.327898472145));
#46121=CARTESIAN_POINT('Ctrl Pts',(-45.3886056079646,-78.2138816873341,
22.5792243900901));
#46122=CARTESIAN_POINT('Ctrl Pts',(-45.2841719635512,-79.7403108235408,
22.3953632331636));
#46123=CARTESIAN_POINT('Ctrl Pts',(-45.1799875089255,-80.9757148217796,
21.6251986126592));
#46124=CARTESIAN_POINT('Ctrl Pts',(-45.0630768128045,-81.7523990234054,
20.0067826286561));
#46125=CARTESIAN_POINT('Ctrl Pts',(-44.9250344935208,-80.8294906995215,
18.0995295298735));
#46126=CARTESIAN_POINT('Ctrl Pts',(-44.8045136744454,-79.1930650736379,
17.4696729318157));
#46127=CARTESIAN_POINT('Ctrl Pts',(-44.701419620499,-77.7364078840939,17.7986961941708));
#46128=CARTESIAN_POINT('Ctrl Pts',(-44.5984229179905,-76.7187699522523,
18.8974867189146));
#46129=CARTESIAN_POINT('Ctrl Pts',(-44.4955825943665,-76.4958138571141,
20.3731005520608));
#46130=CARTESIAN_POINT('Ctrl Pts',(-44.3927708776428,-77.1442359200327,
21.7191405627173));
#46131=CARTESIAN_POINT('Ctrl Pts',(-44.2985803436408,-78.3287975756668,
22.4016406217508));
#46132=CARTESIAN_POINT('Ctrl Pts',(-44.212968657307,-79.5483578860479,22.4006017235312));
#46133=CARTESIAN_POINT('Ctrl Pts',(-44.1359129289841,-80.5369158826798,
21.9250916588476));
#46134=CARTESIAN_POINT('Ctrl Pts',(-44.0716711057434,-81.1071613821891,
21.209794149862));
#46135=CARTESIAN_POINT('Ctrl Pts',(-44.0202796282341,-81.3438226977104,
20.5317985242787));
#46136=CARTESIAN_POINT('Ctrl Pts',(-43.9688671964135,-81.424967756689,19.8178776520423));
#46137=CARTESIAN_POINT('Ctrl Pts',(-43.9045730095602,-81.2211275084576,
18.9256365062025));
#46138=CARTESIAN_POINT('Ctrl Pts',(-43.8273513228911,-80.5359206811645,
18.0651935405777));
#46139=CARTESIAN_POINT('Ctrl Pts',(-43.7500498740938,-79.5443212242324,
17.5887321159173));
#46140=CARTESIAN_POINT('Ctrl Pts',(-43.6597723140765,-78.2581786621976,
17.5864270630418));
#46141=CARTESIAN_POINT('Ctrl Pts',(-43.5563922708837,-76.9708420771708,
18.3903159951276));
#46142=CARTESIAN_POINT('Ctrl Pts',(-43.4397879463254,-76.4046306882061,
20.0093689692673));
#46143=CARTESIAN_POINT('Ctrl Pts',(-43.3228698120996,-76.9711309491329,
21.6305633927173));
#46144=CARTESIAN_POINT('Ctrl Pts',(-43.2055779422275,-78.4300603274151,
22.5488750915416));
#46145=CARTESIAN_POINT('Ctrl Pts',(-43.0878753463866,-80.1489032046835,
22.3562127233884));
#46146=CARTESIAN_POINT('Ctrl Pts',(-42.9697167650604,-81.3775451817227,
21.1294459363969));
#46147=CARTESIAN_POINT('Ctrl Pts',(-42.8510614298393,-81.5740110412663,
19.3969759842311));
#46148=CARTESIAN_POINT('Ctrl Pts',(-42.7318700097782,-80.6433893673584,
17.9132545669706));
#46149=CARTESIAN_POINT('Ctrl Pts',(-42.6121001443425,-78.9824684567483,
17.3306920485745));
#46150=CARTESIAN_POINT('Ctrl Pts',(-42.4917212833099,-77.3125682663215,
17.9134664117972));
#46151=CARTESIAN_POINT('Ctrl Pts',(-42.370679651798,-76.3640214348811,19.4188706488154));
#46152=CARTESIAN_POINT('Ctrl Pts',(-42.2489781115364,-76.5645238873024,
21.1959821363472));
#46153=CARTESIAN_POINT('Ctrl Pts',(-42.1265944138874,-77.8341045341955,
22.4700397556397));
#46154=CARTESIAN_POINT('Ctrl Pts',(-42.0034115172595,-79.6340422101825,
22.6734170894833));
#46155=CARTESIAN_POINT('Ctrl Pts',(-41.9001966362758,-80.9177882354456,
21.8698096826426));
#46156=CARTESIAN_POINT('Ctrl Pts',(-41.817082010737,-81.4823776799116,20.8390969971333));
#46157=CARTESIAN_POINT('Ctrl Pts',(-41.7755178320191,-81.5805519289745,
20.2697706727669));
#46158=CARTESIAN_POINT('Ctrl Pts',(-41.7546186244511,-81.5810972278566,
19.9744962169019));
#46159=CARTESIAN_POINT('Ctrl Pts',(-56.998865393003,-81.8104071381607,19.971749517882));
#46160=CARTESIAN_POINT('Ctrl Pts',(-56.9761215679777,-81.8098137095668,
19.6504133876692));
#46161=CARTESIAN_POINT('Ctrl Pts',(-56.9306422269741,-81.702749946835,19.0272055496801));
#46162=CARTESIAN_POINT('Ctrl Pts',(-56.8393882333594,-81.0832286625891,
17.8952792144066));
#46163=CARTESIAN_POINT('Ctrl Pts',(-56.7246941823819,-79.659154025169,16.9983829421965));
#46164=CARTESIAN_POINT('Ctrl Pts',(-56.5861632252162,-77.6335534097869,
17.2233006398626));
#46165=CARTESIAN_POINT('Ctrl Pts',(-56.4467017882273,-76.1835978989143,
18.6719551219413));
#46166=CARTESIAN_POINT('Ctrl Pts',(-56.3063357852564,-75.9481362494154,
20.7219582178088));
#46167=CARTESIAN_POINT('Ctrl Pts',(-56.1650671343952,-77.0524010984881,
22.4820287706829));
#46168=CARTESIAN_POINT('Ctrl Pts',(-56.022913716882,-79.0240846877592,23.1743286974061));
#46169=CARTESIAN_POINT('Ctrl Pts',(-55.8798883483141,-81.0099417524087,
22.4819069016305));
#46170=CARTESIAN_POINT('Ctrl Pts',(-55.736009170698,-82.1371435389622,20.6919014148508));
#46171=CARTESIAN_POINT('Ctrl Pts',(-55.5912948188564,-81.9011989467447,
18.5773811983794));
#46172=CARTESIAN_POINT('Ctrl Pts',(-55.4457664679998,-80.3895075735084,
17.0631066199702));
#46173=CARTESIAN_POINT('Ctrl Pts',(-55.2994467925014,-78.2525981471427,
16.8201567755944));
#46174=CARTESIAN_POINT('Ctrl Pts',(-55.1523606723563,-76.4194586046196,
17.9695089930655));
#46175=CARTESIAN_POINT('Ctrl Pts',(-55.0291720750146,-75.8221765197523,
19.6778401981353));
#46176=CARTESIAN_POINT('Ctrl Pts',(-54.9302657004888,-76.0582767873485,
21.0517631272575));
#46177=CARTESIAN_POINT('Ctrl Pts',(-54.855911693957,-76.563774636797,21.9689095801494));
#46178=CARTESIAN_POINT('Ctrl Pts',(-54.7813873081152,-77.3470208623382,
22.6677199767267));
#46179=CARTESIAN_POINT('Ctrl Pts',(-54.6817995343713,-78.6425182874698,
23.2077559592215));
#46180=CARTESIAN_POINT('Ctrl Pts',(-54.5569085657542,-80.4660663250115,
23.0055515481889));
#46181=CARTESIAN_POINT('Ctrl Pts',(-54.4064224477222,-82.0323869212294,
21.4408137908159));
#46182=CARTESIAN_POINT('Ctrl Pts',(-54.2553538136249,-82.282138366727,19.2347828818201));
#46183=CARTESIAN_POINT('Ctrl Pts',(-54.1037383696759,-81.0976521492529,
17.3450468644423));
#46184=CARTESIAN_POINT('Ctrl Pts',(-53.9516134654316,-78.9865131673676,
16.6079479997978));
#46185=CARTESIAN_POINT('Ctrl Pts',(-53.799017300736,-76.8685737480114,17.3474746287888));
#46186=CARTESIAN_POINT('Ctrl Pts',(-53.6459896567803,-75.6706931696044,
19.2519276595415));
#46187=CARTESIAN_POINT('Ctrl Pts',(-53.4925710331048,-75.9223549441939,
21.4933728414198));
#46188=CARTESIAN_POINT('Ctrl Pts',(-53.3388026326536,-77.5204065688237,
23.0925152589881));
#46189=CARTESIAN_POINT('Ctrl Pts',(-53.1847265069516,-79.7714109640732,
23.3467986618763));
#46190=CARTESIAN_POINT('Ctrl Pts',(-53.03038548168,-81.6931375902356,22.1399790200489));
#46191=CARTESIAN_POINT('Ctrl Pts',(-52.875823002085,-82.4441600599385,19.9951637320667));
#46192=CARTESIAN_POINT('Ctrl Pts',(-52.7210833439104,-81.6931147568403,
17.847607587344));
#46193=CARTESIAN_POINT('Ctrl Pts',(-52.5662111784277,-79.7652472072559,
16.6359089985643));
#46194=CARTESIAN_POINT('Ctrl Pts',(-52.411251276088,-77.5012356580149,16.8908255535852));
#46195=CARTESIAN_POINT('Ctrl Pts',(-52.256248453475,-75.8897320482582,18.5022380823304));
#46196=CARTESIAN_POINT('Ctrl Pts',(-52.1012476567581,-75.6346189430596,
20.7668255842009));
#46197=CARTESIAN_POINT('Ctrl Pts',(-51.946293812071,-76.8468283649895,22.6957639240306));
#46198=CARTESIAN_POINT('Ctrl Pts',(-51.7914318627055,-78.9959989264195,
23.4475029895662));
#46199=CARTESIAN_POINT('Ctrl Pts',(-51.6367067716067,-81.143023685764,22.6958068198001));
#46200=CARTESIAN_POINT('Ctrl Pts',(-51.4821631962239,-82.3514430242135,
20.7716237421131));
#46201=CARTESIAN_POINT('Ctrl Pts',(-51.3278450629361,-82.0966921870304,
18.5171370441619));
#46202=CARTESIAN_POINT('Ctrl Pts',(-51.173795763927,-80.494660275846,16.9160818675009));
#46203=CARTESIAN_POINT('Ctrl Pts',(-51.0200579736735,-78.2481247248837,
16.6640082062395));
#46204=CARTESIAN_POINT('Ctrl Pts',(-50.8666737295509,-76.3395049302381,
17.8643638570452));
#46205=CARTESIAN_POINT('Ctrl Pts',(-50.713684168159,-75.5963279226902,19.9885708308413));
#46206=CARTESIAN_POINT('Ctrl Pts',(-50.561130291697,-76.3404917399077,22.103826159149));
#46207=CARTESIAN_POINT('Ctrl Pts',(-50.4090511127719,-78.2340315759714,
23.2925880511682));
#46208=CARTESIAN_POINT('Ctrl Pts',(-50.2574850343491,-80.4481760005255,
23.0417916058766));
#46209=CARTESIAN_POINT('Ctrl Pts',(-50.1064690255066,-82.01705159905,21.4708528285098));
#46210=CARTESIAN_POINT('Ctrl Pts',(-49.9560387185426,-82.2630418039423,
19.2728709293431));
#46211=CARTESIAN_POINT('Ctrl Pts',(-49.8062283566168,-81.0898252948096,
17.4088059239318));
#46212=CARTESIAN_POINT('Ctrl Pts',(-49.6570709537323,-79.019024315676,16.68592863221));
#46213=CARTESIAN_POINT('Ctrl Pts',(-49.5085980443133,-76.9595196408508,
17.4088734508976));
#46214=CARTESIAN_POINT('Ctrl Pts',(-49.3608396229039,-75.8040867405457,
19.24850872357));
#46215=CARTESIAN_POINT('Ctrl Pts',(-49.2138236838193,-76.0501675357259,
21.3978373023004));
#46216=CARTESIAN_POINT('Ctrl Pts',(-49.0675767596914,-77.5665861446786,
22.9130985070277));
#46217=CARTESIAN_POINT('Ctrl Pts',(-48.9059614999196,-79.9400679445208,
23.1852360004509));
#46218=CARTESIAN_POINT('Ctrl Pts',(-48.7614602181023,-81.6648094897616,
21.8082179781191));
#46219=CARTESIAN_POINT('Ctrl Pts',(-48.641745504212,-82.0326853928027,20.1333807208566));
#46220=CARTESIAN_POINT('Ctrl Pts',(-48.5622130344089,-81.8465385109611,
19.0326778475393));
#46221=CARTESIAN_POINT('Ctrl Pts',(-48.4670622745342,-81.1987085058851,
17.8562669615047));
#46222=CARTESIAN_POINT('Ctrl Pts',(-48.3486693000866,-79.7268341045547,
16.9318783271684));
#46223=CARTESIAN_POINT('Ctrl Pts',(-48.2074855512855,-77.6628755974866,
17.1663816685728));
#46224=CARTESIAN_POINT('Ctrl Pts',(-48.0672023078574,-76.206752176544,18.626431849987));
#46225=CARTESIAN_POINT('Ctrl Pts',(-47.927830219219,-75.9792981345661,20.6628912290644));
#46226=CARTESIAN_POINT('Ctrl Pts',(-47.7893778161085,-77.0643886294908,
22.3852565245146));
#46227=CARTESIAN_POINT('Ctrl Pts',(-47.6518515237459,-78.9735990241534,
23.0508787165266));
#46228=CARTESIAN_POINT('Ctrl Pts',(-47.5152556014389,-80.8684432520523,
22.3853788812134));
#46229=CARTESIAN_POINT('Ctrl Pts',(-47.3795921088708,-81.9276134623547,
20.6952758178572));
#46230=CARTESIAN_POINT('Ctrl Pts',(-47.2448609079158,-81.7034807862736,
18.7270982413631));
#46231=CARTESIAN_POINT('Ctrl Pts',(-47.1110596886693,-80.3107425715779,
17.3377494473466));
#46232=CARTESIAN_POINT('Ctrl Pts',(-46.9781840026693,-78.3691181398569,
17.1212491527646));
#46233=CARTESIAN_POINT('Ctrl Pts',(-46.8462272430603,-76.7274568500113,
18.1555514656259));
#46234=CARTESIAN_POINT('Ctrl Pts',(-46.7151806507337,-76.0932466642441,
19.9745644839421));
#46235=CARTESIAN_POINT('Ctrl Pts',(-46.5850332874596,-76.72689365866,21.7807592120224));
#46236=CARTESIAN_POINT('Ctrl Pts',(-46.4773155913697,-78.0692304834685,
22.6203028484064));
#46237=CARTESIAN_POINT('Ctrl Pts',(-46.3915770038462,-79.2743999206746,
22.6845333353118));
#46238=CARTESIAN_POINT('Ctrl Pts',(-46.306125933356,-80.4347163011863,22.3540877308873));
#46239=CARTESIAN_POINT('Ctrl Pts',(-46.2140165472685,-81.3855756228331,
21.3981264795911));
#46240=CARTESIAN_POINT('Ctrl Pts',(-46.0871761509613,-81.7920886092443,
19.6302877304961));
#46241=CARTESIAN_POINT('Ctrl Pts',(-45.9979124562317,-81.2080139528857,
18.4010685232934));
#46242=CARTESIAN_POINT('Ctrl Pts',(-45.931706785465,-80.4609863771443,17.8600692258404));
#46243=CARTESIAN_POINT('Ctrl Pts',(-45.8899254264441,-79.9656081265692,
17.5575209097683));
#46244=CARTESIAN_POINT('Ctrl Pts',(-45.8118000032237,-78.880763795498,17.2764338892227));
#46245=CARTESIAN_POINT('Ctrl Pts',(-45.6978306326569,-77.2975836321059,
17.8314065963964));
#46246=CARTESIAN_POINT('Ctrl Pts',(-45.5742396517875,-76.3354201599197,
19.3681907346036));
#46247=CARTESIAN_POINT('Ctrl Pts',(-45.437706343548,-76.5552758080846,21.3715656944865));
#46248=CARTESIAN_POINT('Ctrl Pts',(-45.3020562393531,-78.1821308742347,
22.6659223685449));
#46249=CARTESIAN_POINT('Ctrl Pts',(-45.1941987227426,-79.758928297719,22.475534026443));
#46250=CARTESIAN_POINT('Ctrl Pts',(-45.0866996199815,-81.0338356970261,
21.6807000396746));
#46251=CARTESIAN_POINT('Ctrl Pts',(-44.9662578644687,-81.8333475233177,
20.012518703382));
#46252=CARTESIAN_POINT('Ctrl Pts',(-44.8243750512167,-80.8834891862673,
18.0522457056093));
#46253=CARTESIAN_POINT('Ctrl Pts',(-44.7007996247099,-79.204627825654,17.4066536628875));
#46254=CARTESIAN_POINT('Ctrl Pts',(-44.5952423985192,-77.7129206082217,
17.7439551046314));
#46255=CARTESIAN_POINT('Ctrl Pts',(-44.4900223228441,-76.6730225954323,
18.8674759604783));
#46256=CARTESIAN_POINT('Ctrl Pts',(-44.3851107070103,-76.4459242852341,
20.3731595407077));
#46257=CARTESIAN_POINT('Ctrl Pts',(-44.280478717402,-77.1066399045476,21.7436998539951));
#46258=CARTESIAN_POINT('Ctrl Pts',(-44.1847949217249,-78.3107241896412,
22.4370140832109));
#46259=CARTESIAN_POINT('Ctrl Pts',(-44.0979705969536,-79.5480359338008,
22.4357585099148));
#46260=CARTESIAN_POINT('Ctrl Pts',(-44.0199391969229,-80.5493767638303,
21.9538965049427));
#46261=CARTESIAN_POINT('Ctrl Pts',(-43.9549950707645,-81.1260138276735,
21.230332507434));
#46262=CARTESIAN_POINT('Ctrl Pts',(-43.9030819779796,-81.3650788043183,
20.5453498510557));
#46263=CARTESIAN_POINT('Ctrl Pts',(-43.8511952002441,-81.4469675514213,
19.8246440252031));
#46264=CARTESIAN_POINT('Ctrl Pts',(-43.786381545381,-81.2412693616971,18.9250357363984));
#46265=CARTESIAN_POINT('Ctrl Pts',(-43.7086639057346,-80.5513181773471,
18.058939887935));
#46266=CARTESIAN_POINT('Ctrl Pts',(-43.6309915965552,-79.554575354439,17.5802369898606));
#46267=CARTESIAN_POINT('Ctrl Pts',(-43.5404114400028,-78.2638755524742,
17.5781557379155));
#46268=CARTESIAN_POINT('Ctrl Pts',(-43.4369226415031,-76.9748964799918,
18.3837836136963));
#46269=CARTESIAN_POINT('Ctrl Pts',(-43.3204955018513,-76.409902299744,20.0015897439));
#46270=CARTESIAN_POINT('Ctrl Pts',(-43.2040204721867,-76.9752002181154,
21.6172377254714));
#46271=CARTESIAN_POINT('Ctrl Pts',(-43.0874525410452,-78.4262949071933,
22.5297854402615));
#46272=CARTESIAN_POINT('Ctrl Pts',(-42.9707470684933,-80.1313821068561,
22.3379694555197));
#46273=CARTESIAN_POINT('Ctrl Pts',(-42.8538596468785,-81.3469559099921,
21.1232848086745));
#46274=CARTESIAN_POINT('Ctrl Pts',(-42.7367469025614,-81.5402924255104,
19.4123612569526));
#46275=CARTESIAN_POINT('Ctrl Pts',(-42.6193646471204,-80.6227499332965,
17.950746393619));
#46276=CARTESIAN_POINT('Ctrl Pts',(-42.5016723128577,-78.9894841983059,
17.3785603509998));
#46277=CARTESIAN_POINT('Ctrl Pts',(-42.3836228189166,-77.3512439815465,
17.9509054109146));
#46278=CARTESIAN_POINT('Ctrl Pts',(-42.2651858183516,-76.4228942839963,
19.4252147114051));
#46279=CARTESIAN_POINT('Ctrl Pts',(-42.1462969423314,-76.6193425219703,
21.1617531840419));
#46280=CARTESIAN_POINT('Ctrl Pts',(-42.0269611323496,-77.8579790787978,
22.4041645790426));
#46281=CARTESIAN_POINT('Ctrl Pts',(-41.9070542715169,-79.6104428558897,
22.601547445429));
#46282=CARTESIAN_POINT('Ctrl Pts',(-41.8067886921112,-80.8577927602762,
21.8204122976217));
#46283=CARTESIAN_POINT('Ctrl Pts',(-41.7260879027667,-81.4058116777841,
20.8193752889488));
#46284=CARTESIAN_POINT('Ctrl Pts',(-41.6858137213157,-81.5009183081234,
20.2675948162325));
#46285=CARTESIAN_POINT('Ctrl Pts',(-41.6655045384048,-81.5014482121737,
19.980656523783));
#46286=CARTESIAN_POINT('Ctrl Pts',(-56.9777992245686,-81.7947852592049,
19.6770343419626));
#46287=CARTESIAN_POINT('Ctrl Pts',(-56.9620765160291,-81.7719278227084,
19.4593650843275));
#46288=CARTESIAN_POINT('Ctrl Pts',(-56.923598666368,-81.6549313743044,18.9398363132408));
#46289=CARTESIAN_POINT('Ctrl Pts',(-56.8393882333594,-81.0832286625891,
17.8952792144066));
#46290=CARTESIAN_POINT('Ctrl Pts',(-56.7246941823819,-79.659154025169,16.9983829421965));
#46291=CARTESIAN_POINT('Ctrl Pts',(-56.5861632252162,-77.6335534097869,
17.2233006398626));
#46292=CARTESIAN_POINT('Ctrl Pts',(-56.4467017882273,-76.1835978989143,
18.6719551219413));
#46293=CARTESIAN_POINT('Ctrl Pts',(-56.3063357852564,-75.9481362494154,
20.7219582178088));
#46294=CARTESIAN_POINT('Ctrl Pts',(-56.1650671343952,-77.0524010984881,
22.4820287706829));
#46295=CARTESIAN_POINT('Ctrl Pts',(-56.022913716882,-79.0240846877592,23.1743286974061));
#46296=CARTESIAN_POINT('Ctrl Pts',(-55.8798883483141,-81.0099417524087,
22.4819069016305));
#46297=CARTESIAN_POINT('Ctrl Pts',(-55.736009170698,-82.1371435389622,20.6919014148508));
#46298=CARTESIAN_POINT('Ctrl Pts',(-55.5912948188564,-81.9011989467447,
18.5773811983794));
#46299=CARTESIAN_POINT('Ctrl Pts',(-55.4457664679998,-80.3895075735084,
17.0631066199702));
#46300=CARTESIAN_POINT('Ctrl Pts',(-55.2994467925014,-78.2525981471427,
16.8201567755944));
#46301=CARTESIAN_POINT('Ctrl Pts',(-55.1523606723563,-76.4194586046196,
17.9695089930655));
#46302=CARTESIAN_POINT('Ctrl Pts',(-55.0291720750146,-75.8221765197523,
19.6778401981353));
#46303=CARTESIAN_POINT('Ctrl Pts',(-54.9302657004888,-76.0582767873485,
21.0517631272575));
#46304=CARTESIAN_POINT('Ctrl Pts',(-54.855911693957,-76.563774636797,21.9689095801494));
#46305=CARTESIAN_POINT('Ctrl Pts',(-54.7813873081152,-77.3470208623382,
22.6677199767267));
#46306=CARTESIAN_POINT('Ctrl Pts',(-54.6817995343713,-78.6425182874698,
23.2077559592215));
#46307=CARTESIAN_POINT('Ctrl Pts',(-54.5569085657542,-80.4660663250115,
23.0055515481889));
#46308=CARTESIAN_POINT('Ctrl Pts',(-54.4064224477222,-82.0323869212294,
21.4408137908159));
#46309=CARTESIAN_POINT('Ctrl Pts',(-54.2553538136249,-82.282138366727,19.2347828818201));
#46310=CARTESIAN_POINT('Ctrl Pts',(-54.1037383696759,-81.0976521492529,
17.3450468644423));
#46311=CARTESIAN_POINT('Ctrl Pts',(-53.9516134654316,-78.9865131673676,
16.6079479997978));
#46312=CARTESIAN_POINT('Ctrl Pts',(-53.799017300736,-76.8685737480114,17.3474746287888));
#46313=CARTESIAN_POINT('Ctrl Pts',(-53.6459896567803,-75.6706931696044,
19.2519276595415));
#46314=CARTESIAN_POINT('Ctrl Pts',(-53.4925710331048,-75.9223549441939,
21.4933728414198));
#46315=CARTESIAN_POINT('Ctrl Pts',(-53.3388026326536,-77.5204065688237,
23.0925152589881));
#46316=CARTESIAN_POINT('Ctrl Pts',(-53.1847265069516,-79.7714109640732,
23.3467986618763));
#46317=CARTESIAN_POINT('Ctrl Pts',(-53.03038548168,-81.6931375902356,22.1399790200489));
#46318=CARTESIAN_POINT('Ctrl Pts',(-52.875823002085,-82.4441600599385,19.9951637320667));
#46319=CARTESIAN_POINT('Ctrl Pts',(-52.7210833439104,-81.6931147568403,
17.847607587344));
#46320=CARTESIAN_POINT('Ctrl Pts',(-52.5662111784277,-79.7652472072559,
16.6359089985643));
#46321=CARTESIAN_POINT('Ctrl Pts',(-52.411251276088,-77.5012356580149,16.8908255535852));
#46322=CARTESIAN_POINT('Ctrl Pts',(-52.256248453475,-75.8897320482582,18.5022380823304));
#46323=CARTESIAN_POINT('Ctrl Pts',(-52.1012476567581,-75.6346189430596,
20.7668255842009));
#46324=CARTESIAN_POINT('Ctrl Pts',(-51.946293812071,-76.8468283649895,22.6957639240306));
#46325=CARTESIAN_POINT('Ctrl Pts',(-51.7914318627055,-78.9959989264195,
23.4475029895662));
#46326=CARTESIAN_POINT('Ctrl Pts',(-51.6367067716067,-81.143023685764,22.6958068198001));
#46327=CARTESIAN_POINT('Ctrl Pts',(-51.4821631962239,-82.3514430242135,
20.7716237421131));
#46328=CARTESIAN_POINT('Ctrl Pts',(-51.3278450629361,-82.0966921870304,
18.5171370441619));
#46329=CARTESIAN_POINT('Ctrl Pts',(-51.173795763927,-80.494660275846,16.9160818675009));
#46330=CARTESIAN_POINT('Ctrl Pts',(-51.0200579736735,-78.2481247248837,
16.6640082062395));
#46331=CARTESIAN_POINT('Ctrl Pts',(-50.8666737295509,-76.3395049302381,
17.8643638570452));
#46332=CARTESIAN_POINT('Ctrl Pts',(-50.713684168159,-75.5963279226902,19.9885708308413));
#46333=CARTESIAN_POINT('Ctrl Pts',(-50.561130291697,-76.3404917399077,22.103826159149));
#46334=CARTESIAN_POINT('Ctrl Pts',(-50.4090511127719,-78.2340315759714,
23.2925880511682));
#46335=CARTESIAN_POINT('Ctrl Pts',(-50.2574850343491,-80.4481760005255,
23.0417916058766));
#46336=CARTESIAN_POINT('Ctrl Pts',(-50.1064690255066,-82.01705159905,21.4708528285098));
#46337=CARTESIAN_POINT('Ctrl Pts',(-49.9560387185426,-82.2630418039423,
19.2728709293431));
#46338=CARTESIAN_POINT('Ctrl Pts',(-49.8062283566168,-81.0898252948096,
17.4088059239318));
#46339=CARTESIAN_POINT('Ctrl Pts',(-49.6570709537323,-79.019024315676,16.68592863221));
#46340=CARTESIAN_POINT('Ctrl Pts',(-49.5085980443133,-76.9595196408508,
17.4088734508976));
#46341=CARTESIAN_POINT('Ctrl Pts',(-49.3608396229039,-75.8040867405457,
19.24850872357));
#46342=CARTESIAN_POINT('Ctrl Pts',(-49.2138236838193,-76.0501675357259,
21.3978373023004));
#46343=CARTESIAN_POINT('Ctrl Pts',(-49.0675767596914,-77.5665861446786,
22.9130985070277));
#46344=CARTESIAN_POINT('Ctrl Pts',(-48.9059614999196,-79.9400679445208,
23.1852360004509));
#46345=CARTESIAN_POINT('Ctrl Pts',(-48.7614602181023,-81.6648094897616,
21.8082179781191));
#46346=CARTESIAN_POINT('Ctrl Pts',(-48.641745504212,-82.0326853928027,20.1333807208566));
#46347=CARTESIAN_POINT('Ctrl Pts',(-48.5622130344089,-81.8465385109611,
19.0326778475393));
#46348=CARTESIAN_POINT('Ctrl Pts',(-48.4670622745342,-81.1987085058851,
17.8562669615047));
#46349=CARTESIAN_POINT('Ctrl Pts',(-48.3486693000866,-79.7268341045547,
16.9318783271684));
#46350=CARTESIAN_POINT('Ctrl Pts',(-48.2074855512855,-77.6628755974866,
17.1663816685728));
#46351=CARTESIAN_POINT('Ctrl Pts',(-48.0672023078574,-76.206752176544,18.626431849987));
#46352=CARTESIAN_POINT('Ctrl Pts',(-47.927830219219,-75.9792981345661,20.6628912290644));
#46353=CARTESIAN_POINT('Ctrl Pts',(-47.7893778161085,-77.0643886294908,
22.3852565245146));
#46354=CARTESIAN_POINT('Ctrl Pts',(-47.6518515237459,-78.9735990241534,
23.0508787165266));
#46355=CARTESIAN_POINT('Ctrl Pts',(-47.5152556014389,-80.8684432520523,
22.3853788812134));
#46356=CARTESIAN_POINT('Ctrl Pts',(-47.3795921088708,-81.9276134623547,
20.6952758178572));
#46357=CARTESIAN_POINT('Ctrl Pts',(-47.2448609079158,-81.7034807862736,
18.7270982413631));
#46358=CARTESIAN_POINT('Ctrl Pts',(-47.1110596886693,-80.3107425715779,
17.3377494473466));
#46359=CARTESIAN_POINT('Ctrl Pts',(-46.9781840026693,-78.3691181398569,
17.1212491527646));
#46360=CARTESIAN_POINT('Ctrl Pts',(-46.8462272430603,-76.7274568500113,
18.1555514656259));
#46361=CARTESIAN_POINT('Ctrl Pts',(-46.7151806507337,-76.0932466642441,
19.9745644839421));
#46362=CARTESIAN_POINT('Ctrl Pts',(-46.5850332874596,-76.72689365866,21.7807592120224));
#46363=CARTESIAN_POINT('Ctrl Pts',(-46.4773155913697,-78.0692304834685,
22.6203028484064));
#46364=CARTESIAN_POINT('Ctrl Pts',(-46.3915770038462,-79.2743999206746,
22.6845333353118));
#46365=CARTESIAN_POINT('Ctrl Pts',(-46.306125933356,-80.4347163011863,22.3540877308873));
#46366=CARTESIAN_POINT('Ctrl Pts',(-46.2140165472685,-81.3855756228331,
21.3981264795911));
#46367=CARTESIAN_POINT('Ctrl Pts',(-46.0871761509613,-81.7920886092443,
19.6302877304961));
#46368=CARTESIAN_POINT('Ctrl Pts',(-45.9979124562317,-81.2080139528857,
18.4010685232934));
#46369=CARTESIAN_POINT('Ctrl Pts',(-45.931706785465,-80.4609863771443,17.8600692258404));
#46370=CARTESIAN_POINT('Ctrl Pts',(-45.8899254264441,-79.9656081265692,
17.5575209097683));
#46371=CARTESIAN_POINT('Ctrl Pts',(-45.8118000032237,-78.880763795498,17.2764338892227));
#46372=CARTESIAN_POINT('Ctrl Pts',(-45.6978306326569,-77.2975836321059,
17.8314065963964));
#46373=CARTESIAN_POINT('Ctrl Pts',(-45.5742396517875,-76.3354201599197,
19.3681907346036));
#46374=CARTESIAN_POINT('Ctrl Pts',(-45.437706343548,-76.5552758080846,21.3715656944865));
#46375=CARTESIAN_POINT('Ctrl Pts',(-45.3020562393531,-78.1821308742347,
22.6659223685449));
#46376=CARTESIAN_POINT('Ctrl Pts',(-45.1941987227426,-79.758928297719,22.475534026443));
#46377=CARTESIAN_POINT('Ctrl Pts',(-45.0866996199815,-81.0338356970261,
21.6807000396746));
#46378=CARTESIAN_POINT('Ctrl Pts',(-44.9662578644687,-81.8333475233177,
20.012518703382));
#46379=CARTESIAN_POINT('Ctrl Pts',(-44.8243750512167,-80.8834891862673,
18.0522457056093));
#46380=CARTESIAN_POINT('Ctrl Pts',(-44.7007996247099,-79.204627825654,17.4066536628875));
#46381=CARTESIAN_POINT('Ctrl Pts',(-44.5952423985192,-77.7129206082217,
17.7439551046314));
#46382=CARTESIAN_POINT('Ctrl Pts',(-44.4900223228441,-76.6730225954323,
18.8674759604783));
#46383=CARTESIAN_POINT('Ctrl Pts',(-44.3851107070103,-76.4459242852341,
20.3731595407077));
#46384=CARTESIAN_POINT('Ctrl Pts',(-44.280478717402,-77.1066399045476,21.7436998539951));
#46385=CARTESIAN_POINT('Ctrl Pts',(-44.1847949217249,-78.3107241896412,
22.4370140832109));
#46386=CARTESIAN_POINT('Ctrl Pts',(-44.0979705969536,-79.5480359338008,
22.4357585099148));
#46387=CARTESIAN_POINT('Ctrl Pts',(-44.0199391969229,-80.5493767638303,
21.9538965049427));
#46388=CARTESIAN_POINT('Ctrl Pts',(-43.9549950707645,-81.1260138276735,
21.230332507434));
#46389=CARTESIAN_POINT('Ctrl Pts',(-43.9030819779796,-81.3650788043183,
20.5453498510557));
#46390=CARTESIAN_POINT('Ctrl Pts',(-43.8511952002441,-81.4469675514213,
19.8246440252031));
#46391=CARTESIAN_POINT('Ctrl Pts',(-43.786381545381,-81.2412693616971,18.9250357363984));
#46392=CARTESIAN_POINT('Ctrl Pts',(-43.7086639057346,-80.5513181773471,
18.058939887935));
#46393=CARTESIAN_POINT('Ctrl Pts',(-43.6309915965552,-79.554575354439,17.5802369898606));
#46394=CARTESIAN_POINT('Ctrl Pts',(-43.5404114400028,-78.2638755524742,
17.5781557379155));
#46395=CARTESIAN_POINT('Ctrl Pts',(-43.4369226415031,-76.9748964799918,
18.3837836136963));
#46396=CARTESIAN_POINT('Ctrl Pts',(-43.3204955018513,-76.409902299744,20.0015897439));
#46397=CARTESIAN_POINT('Ctrl Pts',(-43.2040204721867,-76.9752002181154,
21.6172377254714));
#46398=CARTESIAN_POINT('Ctrl Pts',(-43.0874525410452,-78.4262949071933,
22.5297854402615));
#46399=CARTESIAN_POINT('Ctrl Pts',(-42.9707470684933,-80.1313821068561,
22.3379694555197));
#46400=CARTESIAN_POINT('Ctrl Pts',(-42.8538596468785,-81.3469559099921,
21.1232848086745));
#46401=CARTESIAN_POINT('Ctrl Pts',(-42.7367469025614,-81.5402924255104,
19.4123612569526));
#46402=CARTESIAN_POINT('Ctrl Pts',(-42.6193646471204,-80.6227499332965,
17.950746393619));
#46403=CARTESIAN_POINT('Ctrl Pts',(-42.5016723128577,-78.9894841983059,
17.3785603509998));
#46404=CARTESIAN_POINT('Ctrl Pts',(-42.3836228189166,-77.3512439815465,
17.9509054109146));
#46405=CARTESIAN_POINT('Ctrl Pts',(-42.2651858183516,-76.4228942839963,
19.4252147114051));
#46406=CARTESIAN_POINT('Ctrl Pts',(-42.1462969423314,-76.6193425219703,
21.1617531840419));
#46407=CARTESIAN_POINT('Ctrl Pts',(-42.0269611323496,-77.8579790787978,
22.4041645790426));
#46408=CARTESIAN_POINT('Ctrl Pts',(-41.9070542715169,-79.6104428558897,
22.601547445429));
#46409=CARTESIAN_POINT('Ctrl Pts',(-41.8067886921112,-80.8577927602762,
21.8204122976217));
#46410=CARTESIAN_POINT('Ctrl Pts',(-41.7265845261587,-81.4024392322866,
20.8255355557661));
#46411=CARTESIAN_POINT('Ctrl Pts',(-41.6868051036148,-81.4985501065725,
20.281169425713));
#46412=CARTESIAN_POINT('Ctrl Pts',(-41.667003992989,-81.5013236368607,20.0018258382291));
#82348=UNCERTAINTY_MEASURE_WITH_UNIT(LENGTH_MEASURE(0.01),#82385,
'DISTANCE_ACCURACY_VALUE',
'Maximum model space distance between geometric entities at asserted c
onnectivities');
#82363=UNCERTAINTY_MEASURE_WITH_UNIT(LENGTH_MEASURE(0.01),#82385,
'DISTANCE_ACCURACY_VALUE',
'Maximum model space distance between geometric entities at asserted c
onnectivities');
#82369=(
GEOMETRIC_REPRESENTATION_CONTEXT(3)
GLOBAL_UNCERTAINTY_ASSIGNED_CONTEXT((#82348))
GLOBAL_UNIT_ASSIGNED_CONTEXT((#82385,#82387,#82388))
REPRESENTATION_CONTEXT('','3D')
);
#82384=(
GEOMETRIC_REPRESENTATION_CONTEXT(3)
GLOBAL_UNCERTAINTY_ASSIGNED_CONTEXT((#82363))
GLOBAL_UNIT_ASSIGNED_CONTEXT((#82385,#82387,#82388))
REPRESENTATION_CONTEXT('','3D')
);
#82385=(
LENGTH_UNIT()
NAMED_UNIT(*)
SI_UNIT(.MILLI.,.METRE.)
);
#82387=(
NAMED_UNIT(*)
PLANE_ANGLE_UNIT()
SI_UNIT($,.RADIAN.)
);
#82388=(
NAMED_UNIT(*)
SI_UNIT($,.STERADIAN.)
SOLID_ANGLE_UNIT()
);
#82394=SHAPE_DEFINITION_REPRESENTATION(#82414,#82470);
#82414=PRODUCT_DEFINITION_SHAPE('',$,#82491);
#82470=SHAPE_REPRESENTATION('',(#31766),#82369);
#82485=PRODUCT_DEFINITION_CONTEXT('part definition',#82547,'design');
#82491=PRODUCT_DEFINITION('2026-10-20-12-38-29-156',
'16_Rotation_Return_Extension_Spring',#82511,#82485);
#82511=PRODUCT_DEFINITION_FORMATION('',$,#82554);
#82547=APPLICATION_CONTEXT(
'Core Data for Automotive Mechanical Design Process');
#82548=PRODUCT_CONTEXT('part definition',#82547,'mechanical');
#82554=PRODUCT('2026-10-20-12-38-29-156',
'16_Rotation_Return_Extension_Spring',$,(#82548));
#82625=COLOUR_RGB('Grey',0.48,0.52,0.57);
#82626=FILL_AREA_STYLE_COLOUR('',#82625);
#82627=FILL_AREA_STYLE('',(#82626));
#82628=SURFACE_STYLE_FILL_AREA(#82627);
#82629=SURFACE_SIDE_STYLE('',(#82628));
#82630=SURFACE_STYLE_USAGE(.BOTH.,#82629);
#82631=PRESENTATION_STYLE_ASSIGNMENT((#82630));
ENDSEC;
END-ISO-10303-21;
